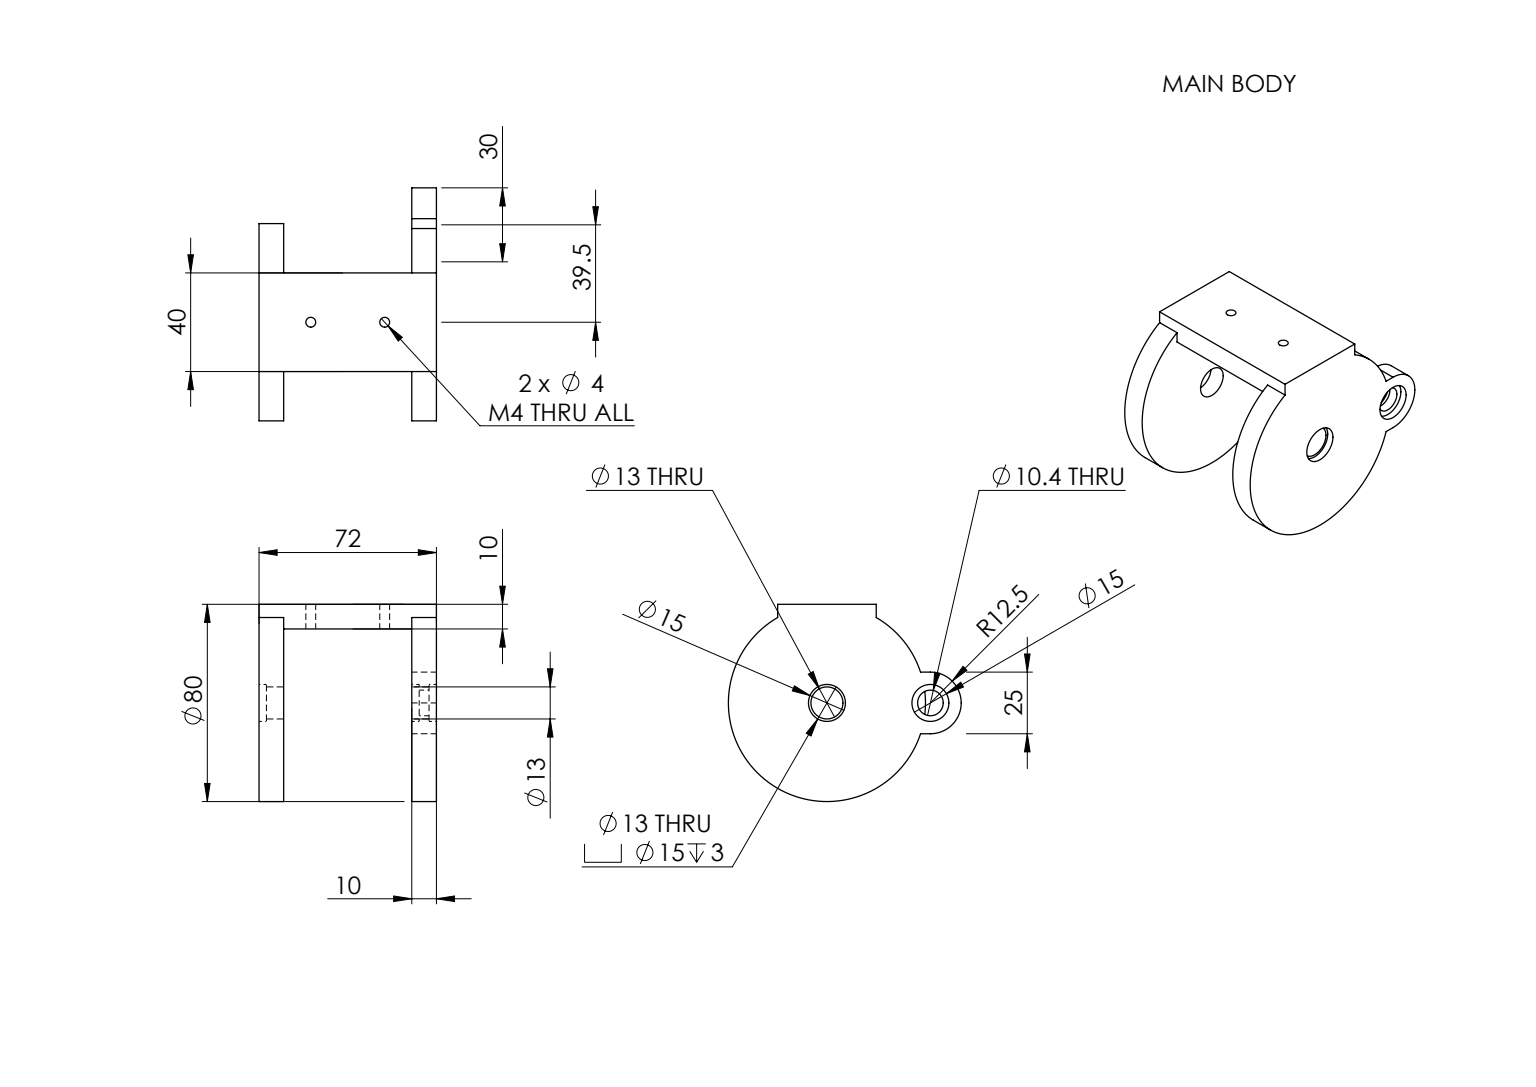
ISO-10303-21;
HEADER;
FILE_DESCRIPTION (('STEP AP214'),
    '1' );
FILE_NAME ('main body.step',
    '2026-10-27T08:02:39',
    ( '' ),
    ( '' ),
    'SwSTEP 2.0',
    'SolidWorks 2026',
    '' );
FILE_SCHEMA (( 'AUTOMOTIVE_DESIGN' ));
ENDSEC;

DATA;
#9=CARTESIAN_POINT ( 'NONE',  ( -36.00100000000000477, 0.000000000000000000, -41.99999999999999289 ) ) ;
#10=ORIENTED_EDGE ( 'NONE', *, *, #7633, .F. ) ;
#14=CIRCLE ( 'NONE', #9018, 40.00000000000000711 ) ;
#19=DIRECTION ( 'NONE',  ( -0.000000000000000000, 1.000000000000000000, -0.000000000000000000 ) ) ;
#37=VECTOR ( 'NONE', #10938, 1000.000000000000000 ) ;
#47=DIRECTION ( 'NONE',  ( 0.000000000000000000, 0.000000000000000000, -1.000000000000000000 ) ) ;
#57=ORIENTED_EDGE ( 'NONE', *, *, #11975, .F. ) ;
#92=DIRECTION ( 'NONE',  ( 1.000000000000000000, -0.000000000000000000, -0.000000000000000000 ) ) ;
#93=CARTESIAN_POINT ( 'NONE',  ( 26.00000000000000355, 0.000000000000000000, -41.99999999999999289 ) ) ;
#96=VECTOR ( 'NONE', #10392, 1000.000000000000000 ) ;
#100=PRODUCT_CONTEXT ( 'NONE', #11984, 'mechanical' ) ;
#103=VERTEX_POINT ( 'NONE', #3228 ) ;
#115=CARTESIAN_POINT ( 'NONE',  ( -26.00000000000000355, -4.898587196589413815E-15, -40.00000000000000711 ) ) ;
#131=CARTESIAN_POINT ( 'NONE',  ( 29.00000000000000000, 9.184850993605147944E-16, -49.49999999999999289 ) ) ;
#146=FACE_OUTER_BOUND ( 'NONE', #6316, .T. ) ;
#153=EDGE_LOOP ( 'NONE', ( #1044, #6924 ) ) ;
#162=DIRECTION ( 'NONE',  ( 1.000000000000000000, 0.000000000000000000, 0.000000000000000000 ) ) ;
#184=DIRECTION ( 'NONE',  ( 1.000000000000000000, 0.000000000000000000, 0.000000000000000000 ) ) ;
#188=CIRCLE ( 'NONE', #6974, 7.500000000000000888 ) ;
#197=CIRCLE ( 'NONE', #11173, 2.000000000000000000 ) ;
#203=CYLINDRICAL_SURFACE ( 'NONE', #8088, 7.500000000000000000 ) ;
#212=CARTESIAN_POINT ( 'NONE',  ( 0.000000000000000000, 0.000000000000000000, 0.000000000000000000 ) ) ;
#213=CIRCLE ( 'NONE', #1019, 7.500000000000000888 ) ;
#231=VERTEX_POINT ( 'NONE', #3477 ) ;
#248=ORIENTED_EDGE ( 'NONE', *, *, #430, .T. ) ;
#256=VECTOR ( 'NONE', #8139, 1000.000000000000000 ) ;
#257=AXIS2_PLACEMENT_3D ( 'NONE', #8422, #11402, #2776 ) ;
#264=ORIENTED_EDGE ( 'NONE', *, *, #11856, .T. ) ;
#278=FACE_OUTER_BOUND ( 'NONE', #10185, .T. ) ;
#294=DIRECTION ( 'NONE',  ( 0.000000000000000000, 0.000000000000000000, -1.000000000000000000 ) ) ;
#297=EDGE_LOOP ( 'NONE', ( #11234, #9949, #2749, #9847 ) ) ;
#298=ORIENTED_EDGE ( 'NONE', *, *, #9479, .T. ) ;
#303=VERTEX_POINT ( 'NONE', #4769 ) ;
#313=MANIFOLD_SOLID_BREP ( 'AdvancedHole1', #9575 ) ;
#315=DIRECTION ( 'NONE',  ( 0.000000000000000000, 0.000000000000000000, -1.000000000000000000 ) ) ;
#322=ORIENTED_EDGE ( 'NONE', *, *, #10069, .T. ) ;
#336=ADVANCED_FACE ( 'NONE', ( #548 ), #10928, .F. ) ;
#387=AXIS2_PLACEMENT_3D ( 'NONE', #11303, #6559, #3504 ) ;
#392=EDGE_LOOP ( 'NONE', ( #8569, #7501, #1729, #4037 ) ) ;
#396=EDGE_CURVE ( 'NONE', #709, #1692, #8083, .T. ) ;
#426=AXIS2_PLACEMENT_3D ( 'NONE', #93, #5779, #1149 ) ;
#429=DIRECTION ( 'NONE',  ( -1.000000000000000000, -0.000000000000000000, -0.000000000000000000 ) ) ;
#430=EDGE_CURVE ( 'NONE', #4941, #709, #2995, .T. ) ;
#433=CARTESIAN_POINT ( 'NONE',  ( 29.00000000000000000, 0.000000000000000000, -34.49999999999999289 ) ) ;
#442=CARTESIAN_POINT ( 'NONE',  ( -26.00000000000000355, 30.00000000000000711, 20.00000000000001066 ) ) ;
#447=EDGE_CURVE ( 'NONE', #1975, #4496, #2545, .T. ) ;
#451=VERTEX_POINT ( 'NONE', #614 ) ;
#483=CARTESIAN_POINT ( 'NONE',  ( 26.00000000000000355, -12.50000000000000000, -37.99671038392666134 ) ) ;
#491=ORIENTED_EDGE ( 'NONE', *, *, #2315, .T. ) ;
#506=SURFACE_STYLE_FILL_AREA ( #8323 ) ;
#508=ORIENTED_EDGE ( 'NONE', *, *, #2896, .F. ) ;
#510=ORIENTED_EDGE ( 'NONE', *, *, #3017, .F. ) ;
#516=CYLINDRICAL_SURFACE ( 'NONE', #1244, 40.00000000000000711 ) ;
#531=FACE_BOUND ( 'NONE', #11009, .T. ) ;
#532=ORIENTED_EDGE ( 'NONE', *, *, #567, .F. ) ;
#548=FACE_OUTER_BOUND ( 'NONE', #392, .T. ) ;
#550=DIRECTION ( 'NONE',  ( 0.000000000000000000, 0.000000000000000000, 1.000000000000000000 ) ) ;
#552=FACE_BOUND ( 'NONE', #153, .T. ) ;
#567=EDGE_CURVE ( 'NONE', #11902, #11981, #6636, .T. ) ;
#571=DIRECTION ( 'NONE',  ( 1.000000000000000000, -0.000000000000000000, -0.000000000000000000 ) ) ;
#572=AXIS2_PLACEMENT_3D ( 'NONE', #11910, #10065, #680 ) ;
#589=LINE ( 'NONE', #3484, #11033 ) ;
#591=CARTESIAN_POINT ( 'NONE',  ( 36.00000000000000711, 0.000000000000000000, -41.99999999999999289 ) ) ;
#596=AXIS2_PLACEMENT_3D ( 'NONE', #7195, #3371, #9943 ) ;
#598=CARTESIAN_POINT ( 'NONE',  ( 33.00000000000000000, 0.000000000000000000, 0.000000000000000000 ) ) ;
#603=AXIS2_PLACEMENT_3D ( 'NONE', #7936, #5992, #9880 ) ;
#614=CARTESIAN_POINT ( 'NONE',  ( 33.00000000000000000, 0.000000000000000000, -47.19999999999998863 ) ) ;
#657=DIRECTION ( 'NONE',  ( 1.000000000000000000, 0.000000000000000000, 0.000000000000000000 ) ) ;
#663=ADVANCED_FACE ( 'NONE', ( #9634 ), #5938, .T. ) ;
#664=DIRECTION ( 'NONE',  ( -0.000000000000000000, 1.000000000000000000, -0.000000000000000000 ) ) ;
#680=DIRECTION ( 'NONE',  ( 0.000000000000000000, 0.000000000000000000, -1.000000000000000000 ) ) ;
#682=CARTESIAN_POINT ( 'NONE',  ( 36.00000000000000711, 34.64101615137756340, -19.99999999999998934 ) ) ;
#688=DIRECTION ( 'NONE',  ( 0.000000000000000000, -0.000000000000000000, 1.000000000000000000 ) ) ;
#689=PLANE ( 'NONE',  #1651 ) ;
#691=ORIENTED_EDGE ( 'NONE', *, *, #7322, .T. ) ;
#704=LINE ( 'NONE', #8215, #4042 ) ;
#709=VERTEX_POINT ( 'NONE', #9052 ) ;
#726=CARTESIAN_POINT ( 'NONE',  ( 26.00000000000000355, 0.000000000000000000, 0.000000000000000000 ) ) ;
#735=ORIENTED_EDGE ( 'NONE', *, *, #8854, .T. ) ;
#739=FACE_OUTER_BOUND ( 'NONE', #4011, .T. ) ;
#741=EDGE_LOOP ( 'NONE', ( #2743, #11355 ) ) ;
#754=DIRECTION ( 'NONE',  ( -1.000000000000000000, -0.000000000000000000, -0.000000000000000000 ) ) ;
#755=ORIENTED_EDGE ( 'NONE', *, *, #1742, .T. ) ;
#780=FACE_OUTER_BOUND ( 'NONE', #2241, .T. ) ;
#790=EDGE_CURVE ( 'NONE', #1934, #9986, #4294, .T. ) ;
#794=FACE_OUTER_BOUND ( 'NONE', #9487, .T. ) ;
#807=EDGE_CURVE ( 'NONE', #5230, #2486, #7399, .T. ) ;
#825=VERTEX_POINT ( 'NONE', #483 ) ;
#829=EDGE_LOOP ( 'NONE', ( #5890, #10432, #3205, #5681, #3589, #1932, #7496, #8486 ) ) ;
#837=VECTOR ( 'NONE', #8894, 1000.000000000000000 ) ;
#842=DIRECTION ( 'NONE',  ( 1.000000000000000000, -0.000000000000000000, -0.000000000000000000 ) ) ;
#843=LINE ( 'NONE', #5480, #11789 ) ;
#844=ORIENTED_EDGE ( 'NONE', *, *, #6702, .F. ) ;
#903=DIRECTION ( 'NONE',  ( 1.000000000000000000, -0.000000000000000000, -0.000000000000000000 ) ) ;
#912=EDGE_LOOP ( 'NONE', ( #4953, #8523 ) ) ;
#921=DIRECTION ( 'NONE',  ( 1.000000000000000000, 0.000000000000000000, 0.000000000000000000 ) ) ;
#959=ORIENTED_EDGE ( 'NONE', *, *, #12102, .F. ) ;
#964=DIRECTION ( 'NONE',  ( 0.000000000000000000, 0.000000000000000000, 1.000000000000000000 ) ) ;
#969=CARTESIAN_POINT ( 'NONE',  ( 29.00000000000000000, 0.000000000000000000, -41.99999999999999289 ) ) ;
#971=VECTOR ( 'NONE', #6375, 1000.000000000000000 ) ;
#977=CARTESIAN_POINT ( 'NONE',  ( 33.00000000000000000, 0.000000000000000000, 0.000000000000000000 ) ) ;
#983=ORIENTED_EDGE ( 'NONE', *, *, #11550, .F. ) ;
#1000=CARTESIAN_POINT ( 'NONE',  ( 36.00000000000000711, 0.000000000000000000, 0.000000000000000000 ) ) ;
#1019=AXIS2_PLACEMENT_3D ( 'NONE', #11811, #1311, #7951 ) ;
#1035=VECTOR ( 'NONE', #1350, 1000.000000000000000 ) ;
#1044=ORIENTED_EDGE ( 'NONE', *, *, #4471, .F. ) ;
#1051=EDGE_CURVE ( 'NONE', #9332, #5880, #9739, .T. ) ;
#1065=DIRECTION ( 'NONE',  ( 0.000000000000000000, 0.000000000000000000, 1.000000000000000000 ) ) ;
#1089=AXIS2_PLACEMENT_3D ( 'NONE', #3095, #10765, #8031 ) ;
#1096=CIRCLE ( 'NONE', #10089, 12.49999999999999645 ) ;
#1126=CARTESIAN_POINT ( 'NONE',  ( 26.00000000000000355, 0.000000000000000000, -41.99999999999999289 ) ) ;
#1128=ORIENTED_EDGE ( 'NONE', *, *, #8084, .T. ) ;
#1149=DIRECTION ( 'NONE',  ( 0.000000000000000000, 0.000000000000000000, 1.000000000000000000 ) ) ;
#1151=ORIENTED_EDGE ( 'NONE', *, *, #2334, .F. ) ;
#1152=DIRECTION ( 'NONE',  ( 0.000000000000000000, 1.000000000000000000, 0.000000000000000000 ) ) ;
#1156=CARTESIAN_POINT ( 'NONE',  ( -26.00000000000000355, 0.000000000000000000, 0.000000000000000000 ) ) ;
#1164=AXIS2_PLACEMENT_3D ( 'NONE', #1603, #3421, #7254 ) ;
#1166=CIRCLE ( 'NONE', #8970, 12.49999999999999645 ) ;
#1198=DIRECTION ( 'NONE',  ( -0.000000000000000000, 1.000000000000000000, -0.000000000000000000 ) ) ;
#1215=CARTESIAN_POINT ( 'NONE',  ( 26.00000000000000355, 7.960204194457796463E-16, -6.500000000000000888 ) ) ;
#1218=VECTOR ( 'NONE', #8496, 1000.000000000000000 ) ;
#1220=ORIENTED_EDGE ( 'NONE', *, *, #12267, .F. ) ;
#1232=ORIENTED_EDGE ( 'NONE', *, *, #5271, .T. ) ;
#1244=AXIS2_PLACEMENT_3D ( 'NONE', #11020, #571, #5466 ) ;
#1248=LINE ( 'NONE', #5066, #837 ) ;
#1271=CARTESIAN_POINT ( 'NONE',  ( -36.00000000000000711, 0.000000000000000000, 0.000000000000000000 ) ) ;
#1288=CIRCLE ( 'NONE', #1089, 40.00000000000000711 ) ;
#1298=AXIS2_PLACEMENT_3D ( 'NONE', #8826, #184, #9826 ) ;
#1299=CARTESIAN_POINT ( 'NONE',  ( 33.00000000000000000, 9.184850993605149917E-16, 7.500000000000000888 ) ) ;
#1304=CARTESIAN_POINT ( 'NONE',  ( -36.00000000000000000, 40.00000000000000711, 20.00000000000001066 ) ) ;
#1311=DIRECTION ( 'NONE',  ( 1.000000000000000000, 0.000000000000000000, 0.000000000000000000 ) ) ;
#1315=EDGE_LOOP ( 'NONE', ( #8246, #5545, #4189, #9435 ) ) ;
#1317=EDGE_CURVE ( 'NONE', #2662, #10589, #3298, .T. ) ;
#1320=VERTEX_POINT ( 'NONE', #4590 ) ;
#1325=CARTESIAN_POINT ( 'NONE',  ( -36.00000000000000711, 0.000000000000000000, 6.500000000000000888 ) ) ;
#1328=CARTESIAN_POINT ( 'NONE',  ( 26.00000000000000355, 12.50000000000000000, -24.50000000000000000 ) ) ;
#1329=ORIENTED_EDGE ( 'NONE', *, *, #10497, .T. ) ;
#1331=CARTESIAN_POINT ( 'NONE',  ( -26.00000000000000355, 34.64101615137756340, -19.99999999999998934 ) ) ;
#1341=CARTESIAN_POINT ( 'NONE',  ( -15.00000000000000000, 40.00000000000000711, -2.000000000000000000 ) ) ;
#1350=DIRECTION ( 'NONE',  ( 1.000000000000000000, -0.000000000000000000, -0.000000000000000000 ) ) ;
#1363=LINE ( 'NONE', #433, #6985 ) ;
#1395=ORIENTED_EDGE ( 'NONE', *, *, #8716, .F. ) ;
#1397=EDGE_CURVE ( 'NONE', #8903, #2114, #6531, .T. ) ;
#1417=CIRCLE ( 'NONE', #11191, 40.00000000000000711 ) ;
#1424=VERTEX_POINT ( 'NONE', #11327 ) ;
#1427=COLOUR_RGB ( '',0.8941176470588234615, 0.8941176470588234615, 0.8941176470588234615 ) ;
#1434=CARTESIAN_POINT ( 'NONE',  ( -36.00000000000000711, 34.64101615137756340, -19.99999999999998934 ) ) ;
#1437=ADVANCED_FACE ( 'NONE', ( #10586, #10331 ), #8536, .T. ) ;
#1447=LINE ( 'NONE', #442, #256 ) ;
#1468=CARTESIAN_POINT ( 'NONE',  ( 36.00000000000000000, 30.00000000000000711, -19.99999999999998934 ) ) ;
#1478=DIRECTION ( 'NONE',  ( -1.000000000000000000, 0.000000000000000000, 0.000000000000000000 ) ) ;
#1485=ADVANCED_FACE ( 'NONE', ( #146 ), #1910, .F. ) ;
#1489=LINE ( 'NONE', #9124, #6369 ) ;
#1491=VERTEX_POINT ( 'NONE', #7725 ) ;
#1494=VERTEX_POINT ( 'NONE', #6594 ) ;
#1504=CARTESIAN_POINT ( 'NONE',  ( 29.00000000000000000, 0.000000000000000000, -41.99999999999999289 ) ) ;
#1505=DIRECTION ( 'NONE',  ( 1.000000000000000000, 0.000000000000000000, 0.000000000000000000 ) ) ;
#1511=CARTESIAN_POINT ( 'NONE',  ( 26.00000000000000355, 0.000000000000000000, 0.000000000000000000 ) ) ;
#1521=CARTESIAN_POINT ( 'NONE',  ( 36.00000000000000711, 0.000000000000000000, 40.00000000000000711 ) ) ;
#1522=LINE ( 'NONE', #9285, #12208 ) ;
#1535=DIRECTION ( 'NONE',  ( -0.000000000000000000, 1.000000000000000000, 0.000000000000000000 ) ) ;
#1542=ORIENTED_EDGE ( 'NONE', *, *, #447, .F. ) ;
#1547=ORIENTED_EDGE ( 'NONE', *, *, #4092, .F. ) ;
#1550=ORIENTED_EDGE ( 'NONE', *, *, #10879, .T. ) ;
#1571=EDGE_CURVE ( 'NONE', #9332, #4951, #6562, .T. ) ;
#1589=CARTESIAN_POINT ( 'NONE',  ( 26.00000000000000355, 34.64101615137754919, 20.00000000000000711 ) ) ;
#1594=FACE_OUTER_BOUND ( 'NONE', #8873, .T. ) ;
#1603=CARTESIAN_POINT ( 'NONE',  ( -13.05124837953327344, 0.000000000000000000, -41.99999999999999289 ) ) ;
#1605=ORIENTED_EDGE ( 'NONE', *, *, #9074, .T. ) ;
#1637=AXIS2_PLACEMENT_3D ( 'NONE', #7596, #92, #6914 ) ;
#1639=AXIS2_PLACEMENT_3D ( 'NONE', #1955, #4829, #8652 ) ;
#1651=AXIS2_PLACEMENT_3D ( 'NONE', #7383, #12110, #6376 ) ;
#1655=UNCERTAINTY_MEASURE_WITH_UNIT (LENGTH_MEASURE( 1.000000000000000082E-05 ), #6454, 'distance_accuracy_value', 'NONE');
#1665=CARTESIAN_POINT ( 'NONE',  ( 28.99999999999999645, 6.368163355566238354E-16, -36.79999999999999716 ) ) ;
#1684=CARTESIAN_POINT ( 'NONE',  ( -36.00100000000000477, 0.000000000000000000, -47.19999999999998863 ) ) ;
#1686=VERTEX_POINT ( 'NONE', #3101 ) ;
#1692=VERTEX_POINT ( 'NONE', #2092 ) ;
#1694=( NAMED_UNIT ( * ) PLANE_ANGLE_UNIT ( ) SI_UNIT ( $, .RADIAN. ) );
#1697=ORIENTED_EDGE ( 'NONE', *, *, #7444, .T. ) ;
#1709=VERTEX_POINT ( 'NONE', #9858 ) ;
#1721=ORIENTED_EDGE ( 'NONE', *, *, #7312, .T. ) ;
#1729=ORIENTED_EDGE ( 'NONE', *, *, #7563, .F. ) ;
#1742=EDGE_CURVE ( 'NONE', #8475, #303, #4087, .T. ) ;
#1752=CARTESIAN_POINT ( 'NONE',  ( 26.00000000000000355, 0.000000000000000000, -41.99999999999999289 ) ) ;
#1758=ORIENTED_EDGE ( 'NONE', *, *, #10893, .F. ) ;
#1761=ORIENTED_EDGE ( 'NONE', *, *, #2117, .F. ) ;
#1776=CARTESIAN_POINT ( 'NONE',  ( 36.00000000000000711, 0.000000000000000000, 0.000000000000000000 ) ) ;
#1790=FACE_BOUND ( 'NONE', #2715, .T. ) ;
#1796=DIRECTION ( 'NONE',  ( 0.000000000000000000, 0.000000000000000000, 1.000000000000000000 ) ) ;
#1806=DIRECTION ( 'NONE',  ( 1.000000000000000000, -0.000000000000000000, -0.000000000000000000 ) ) ;
#1810=DIRECTION ( 'NONE',  ( -0.000000000000000000, 1.000000000000000000, 0.000000000000000000 ) ) ;
#1813=ORIENTED_EDGE ( 'NONE', *, *, #6114, .F. ) ;
#1825=AXIS2_PLACEMENT_3D ( 'NONE', #7929, #9873, #6296 ) ;
#1838=ORIENTED_EDGE ( 'NONE', *, *, #396, .T. ) ;
#1840=CIRCLE ( 'NONE', #2837, 7.500000000000000000 ) ;
#1861=AXIS2_PLACEMENT_3D ( 'NONE', #4094, #10529, #7862 ) ;
#1863=CARTESIAN_POINT ( 'NONE',  ( 26.00000000000000355, 0.000000000000000000, 0.000000000000000000 ) ) ;
#1869=ADVANCED_FACE ( 'NONE', ( #5394 ), #11081, .F. ) ;
#1872=DIRECTION ( 'NONE',  ( 0.000000000000000000, 0.000000000000000000, -1.000000000000000000 ) ) ;
#1874=EDGE_LOOP ( 'NONE', ( #1935, #4316, #491, #959 ) ) ;
#1877=DIRECTION ( 'NONE',  ( 1.000000000000000000, -0.000000000000000000, -0.000000000000000000 ) ) ;
#1878=CARTESIAN_POINT ( 'NONE',  ( 36.00000000000000711, 0.000000000000000000, 0.000000000000000000 ) ) ;
#1910=PLANE ( 'NONE',  #2966 ) ;
#1925=FACE_BOUND ( 'NONE', #6583, .T. ) ;
#1932=ORIENTED_EDGE ( 'NONE', *, *, #3099, .T. ) ;
#1934=VERTEX_POINT ( 'NONE', #6518 ) ;
#1935=ORIENTED_EDGE ( 'NONE', *, *, #12053, .F. ) ;
#1938=CARTESIAN_POINT ( 'NONE',  ( -36.00100000000000477, 0.000000000000000000, -41.99999999999999289 ) ) ;
#1941=CARTESIAN_POINT ( 'NONE',  ( 26.00000000000000355, 0.000000000000000000, 6.500000000000000888 ) ) ;
#1955=CARTESIAN_POINT ( 'NONE',  ( -13.05124837953327344, -12.50000000000000000, -24.50000000000000000 ) ) ;
#1975=VERTEX_POINT ( 'NONE', #10511 ) ;
#2015=AXIS2_PLACEMENT_3D ( 'NONE', #4944, #11557, #3087 ) ;
#2033=DIRECTION ( 'NONE',  ( 0.000000000000000000, 0.000000000000000000, -1.000000000000000000 ) ) ;
#2053=DIRECTION ( 'NONE',  ( 1.000000000000000000, -0.000000000000000000, -0.000000000000000000 ) ) ;
#2056=DIRECTION ( 'NONE',  ( 1.000000000000000000, -0.000000000000000000, -0.000000000000000000 ) ) ;
#2062=DIRECTION ( 'NONE',  ( 1.000000000000000000, 0.000000000000000000, -0.000000000000000000 ) ) ;
#2073=CYLINDRICAL_SURFACE ( 'NONE', #12012, 7.500000000000000888 ) ;
#2082=CARTESIAN_POINT ( 'NONE',  ( -36.00000000000000711, -9.184850993605149917E-16, 7.500000000000000888 ) ) ;
#2085=CYLINDRICAL_SURFACE ( 'NONE', #4823, 5.199999999999996625 ) ;
#2092=CARTESIAN_POINT ( 'NONE',  ( 36.00000000000000711, 0.000000000000000000, -49.49999999999999289 ) ) ;
#2108=FACE_OUTER_BOUND ( 'NONE', #4777, .T. ) ;
#2109=ORIENTED_EDGE ( 'NONE', *, *, #10098, .T. ) ;
#2114=VERTEX_POINT ( 'NONE', #4185 ) ;
#2117=EDGE_CURVE ( 'NONE', #1320, #10764, #7211, .T. ) ;
#2129=ORIENTED_EDGE ( 'NONE', *, *, #1571, .F. ) ;
#2140=EDGE_CURVE ( 'NONE', #1975, #825, #8952, .T. ) ;
#2147=VERTEX_POINT ( 'NONE', #9768 ) ;
#2157=FACE_OUTER_BOUND ( 'NONE', #6571, .T. ) ;
#2159=ORIENTED_EDGE ( 'NONE', *, *, #4246, .T. ) ;
#2160=ORIENTED_EDGE ( 'NONE', *, *, #11856, .F. ) ;
#2166=ORIENTED_EDGE ( 'NONE', *, *, #2958, .T. ) ;
#2173=ADVANCED_FACE ( 'NONE', ( #11347, #10011 ), #2366, .T. ) ;
#2182=ADVANCED_FACE ( 'NONE', ( #10930 ), #4253, .F. ) ;
#2190=LINE ( 'NONE', #6129, #10988 ) ;
#2241=EDGE_LOOP ( 'NONE', ( #1761, #9174, #4530, #6960 ) ) ;
#2243=CARTESIAN_POINT ( 'NONE',  ( 36.00000000000000711, 0.000000000000000000, -54.50000000000000000 ) ) ;
#2249=ORIENTED_EDGE ( 'NONE', *, *, #10231, .T. ) ;
#2252=VECTOR ( 'NONE', #11067, 1000.000000000000000 ) ;
#2281=CIRCLE ( 'NONE', #7082, 1.999999999999998224 ) ;
#2298=VERTEX_POINT ( 'NONE', #8617 ) ;
#2303=LINE ( 'NONE', #1434, #5639 ) ;
#2311=FACE_BOUND ( 'NONE', #10416, .T. ) ;
#2315=EDGE_CURVE ( 'NONE', #2452, #10319, #7420, .T. ) ;
#2334=EDGE_CURVE ( 'NONE', #1494, #3376, #2866, .T. ) ;
#2354=ADVANCED_FACE ( 'NONE', ( #3923, #2108 ), #9552, .T. ) ;
#2362=CARTESIAN_POINT ( 'NONE',  ( 26.00000000000000355, 12.50000000000000000, -41.99999999999999289 ) ) ;
#2366=PLANE ( 'NONE',  #2407 ) ;
#2383=CIRCLE ( 'NONE', #7794, 12.49999999999999645 ) ;
#2386=CIRCLE ( 'NONE', #5753, 7.500000000000000888 ) ;
#2392=CYLINDRICAL_SURFACE ( 'NONE', #5568, 7.500000000000000000 ) ;
#2394=ORIENTED_EDGE ( 'NONE', *, *, #8102, .F. ) ;
#2400=CARTESIAN_POINT ( 'NONE',  ( -15.00000000000000000, 30.00000000000000711, 0.000000000000000000 ) ) ;
#2407=AXIS2_PLACEMENT_3D ( 'NONE', #1504, #11118, #550 ) ;
#2418=AXIS2_PLACEMENT_3D ( 'NONE', #977, #921, #47 ) ;
#2422=EDGE_CURVE ( 'NONE', #303, #11981, #4418, .T. ) ;
#2426=VERTEX_POINT ( 'NONE', #12345 ) ;
#2429=CYLINDRICAL_SURFACE ( 'NONE', #9502, 7.500000000000000000 ) ;
#2432=EDGE_CURVE ( 'NONE', #6862, #5581, #14, .T. ) ;
#2440=LINE ( 'NONE', #8318, #2252 ) ;
#2450=CIRCLE ( 'NONE', #6624, 5.199999999999996625 ) ;
#2452=VERTEX_POINT ( 'NONE', #1341 ) ;
#2457=CIRCLE ( 'NONE', #6260, 7.500000000000000000 ) ;
#2461=CARTESIAN_POINT ( 'NONE',  ( -13.05124837953327344, 12.50000000000000000, -41.99999999999999289 ) ) ;
#2463=ORIENTED_EDGE ( 'NONE', *, *, #7322, .F. ) ;
#2479=ORIENTED_EDGE ( 'NONE', *, *, #7267, .F. ) ;
#2482=CARTESIAN_POINT ( 'NONE',  ( 36.00000000000000000, 40.00000000000000711, 20.00000000000001066 ) ) ;
#2486=VERTEX_POINT ( 'NONE', #10786 ) ;
#2545=LINE ( 'NONE', #3558, #10976 ) ;
#2547=DIRECTION ( 'NONE',  ( -0.000000000000000000, 1.000000000000000000, -0.000000000000000000 ) ) ;
#2548=EDGE_CURVE ( 'NONE', #4639, #4147, #10908, .T. ) ;
#2551=DIRECTION ( 'NONE',  ( 1.000000000000000000, -0.000000000000000000, -0.000000000000000000 ) ) ;
#2552=ADVANCED_FACE ( 'NONE', ( #531, #2157 ), #5048, .T. ) ;
#2553=EDGE_LOOP ( 'NONE', ( #8988, #1128, #7779, #7206, #2918, #2166, #691, #2249, #9046, #2109 ) ) ;
#2556=( LENGTH_UNIT ( ) NAMED_UNIT ( * ) SI_UNIT ( .MILLI., .METRE. ) );
#2567=DIRECTION ( 'NONE',  ( 0.000000000000000000, -0.000000000000000000, 1.000000000000000000 ) ) ;
#2570=APPLICATION_CONTEXT ( 'automotive_design' ) ;
#2581=EDGE_CURVE ( 'NONE', #6339, #1692, #5417, .T. ) ;
#2625=( NAMED_UNIT ( * ) SI_UNIT ( $, .STERADIAN. ) SOLID_ANGLE_UNIT ( ) );
#2629=EDGE_LOOP ( 'NONE', ( #11526, #3927, #5490, #12163 ) ) ;
#2641=FACE_OUTER_BOUND ( 'NONE', #297, .T. ) ;
#2642=AXIS2_PLACEMENT_3D ( 'NONE', #1000, #9706, #8757 ) ;
#2651=EDGE_CURVE ( 'NONE', #2486, #4605, #843, .T. ) ;
#2659=LINE ( 'NONE', #5589, #9831 ) ;
#2661=VERTEX_POINT ( 'NONE', #1665 ) ;
#2662=VERTEX_POINT ( 'NONE', #9300 ) ;
#2675=DIRECTION ( 'NONE',  ( 1.000000000000000000, 0.000000000000000000, 0.000000000000000000 ) ) ;
#2676=ORIENTED_EDGE ( 'NONE', *, *, #2117, .T. ) ;
#2688=ORIENTED_EDGE ( 'NONE', *, *, #7992, .T. ) ;
#2715=EDGE_LOOP ( 'NONE', ( #9455, #9983 ) ) ;
#2722=DIRECTION ( 'NONE',  ( 1.000000000000000000, 0.000000000000000000, 0.000000000000000000 ) ) ;
#2743=ORIENTED_EDGE ( 'NONE', *, *, #8913, .T. ) ;
#2748=DIRECTION ( 'NONE',  ( -1.000000000000000000, -0.000000000000000000, -0.000000000000000000 ) ) ;
#2749=ORIENTED_EDGE ( 'NONE', *, *, #10679, .F. ) ;
#2758=CARTESIAN_POINT ( 'NONE',  ( -33.00000000000000000, 0.000000000000000000, 0.000000000000000000 ) ) ;
#2764=EDGE_LOOP ( 'NONE', ( #1329, #2839 ) ) ;
#2776=DIRECTION ( 'NONE',  ( 0.000000000000000000, 0.000000000000000000, 1.000000000000000000 ) ) ;
#2803=EDGE_CURVE ( 'NONE', #1424, #1709, #5830, .T. ) ;
#2821=AXIS2_PLACEMENT_3D ( 'NONE', #4721, #664, #7600 ) ;
#2834=AXIS2_PLACEMENT_3D ( 'NONE', #1776, #9482, #5412 ) ;
#2836=DIRECTION ( 'NONE',  ( 0.000000000000000000, 0.000000000000000000, -1.000000000000000000 ) ) ;
#2837=AXIS2_PLACEMENT_3D ( 'NONE', #1126, #10446, #4937 ) ;
#2838=VECTOR ( 'NONE', #10774, 1000.000000000000000 ) ;
#2839=ORIENTED_EDGE ( 'NONE', *, *, #4092, .T. ) ;
#2844=CARTESIAN_POINT ( 'NONE',  ( -33.00000000000000000, 0.000000000000000000, 6.500000000000000888 ) ) ;
#2851=CYLINDRICAL_SURFACE ( 'NONE', #257, 6.500000000000000888 ) ;
#2866=LINE ( 'NONE', #3979, #11990 ) ;
#2877=CARTESIAN_POINT ( 'NONE',  ( 15.00000000000000355, 40.00000000000000711, 1.999999999999998224 ) ) ;
#2887=FACE_OUTER_BOUND ( 'NONE', #5644, .T. ) ;
#2890=DIRECTION ( 'NONE',  ( 0.000000000000000000, 0.000000000000000000, -1.000000000000000000 ) ) ;
#2896=EDGE_CURVE ( 'NONE', #1494, #9332, #8834, .T. ) ;
#2900=DIRECTION ( 'NONE',  ( 0.000000000000000000, 0.000000000000000000, 1.000000000000000000 ) ) ;
#2918=ORIENTED_EDGE ( 'NONE', *, *, #2432, .T. ) ;
#2923=CARTESIAN_POINT ( 'NONE',  ( 33.00000000000000000, 0.000000000000000000, -41.99999999999999289 ) ) ;
#2924=DIRECTION ( 'NONE',  ( 0.000000000000000000, 0.000000000000000000, -1.000000000000000000 ) ) ;
#2935=ADVANCED_FACE ( 'NONE', ( #278 ), #9789, .F. ) ;
#2936=FACE_BOUND ( 'NONE', #912, .T. ) ;
#2939=CARTESIAN_POINT ( 'NONE',  ( 26.00000000000000355, 0.000000000000000000, 0.000000000000000000 ) ) ;
#2941=CYLINDRICAL_SURFACE ( 'NONE', #6493, 6.500000000000000888 ) ;
#2958=EDGE_CURVE ( 'NONE', #5581, #10639, #4203, .T. ) ;
#2966=AXIS2_PLACEMENT_3D ( 'NONE', #12321, #10399, #11576 ) ;
#2995=CIRCLE ( 'NONE', #387, 7.500000000000000000 ) ;
#3014=CARTESIAN_POINT ( 'NONE',  ( -26.00000000000000355, 30.00000000000000711, 20.00000000000001066 ) ) ;
#3017=EDGE_CURVE ( 'NONE', #8676, #6734, #3104, .T. ) ;
#3024=ORIENTED_EDGE ( 'NONE', *, *, #4423, .F. ) ;
#3062=AXIS2_PLACEMENT_3D ( 'NONE', #11201, #7341, #2567 ) ;
#3085=LINE ( 'NONE', #9764, #8389 ) ;
#3087=DIRECTION ( 'NONE',  ( 0.000000000000000000, 0.000000000000000000, 1.000000000000000000 ) ) ;
#3093=CARTESIAN_POINT ( 'NONE',  ( -15.00000000000000000, 40.00000000000000711, 0.000000000000000000 ) ) ;
#3094=ORIENTED_EDGE ( 'NONE', *, *, #2896, .T. ) ;
#3095=CARTESIAN_POINT ( 'NONE',  ( -26.00000000000000355, 0.000000000000000000, 0.000000000000000000 ) ) ;
#3099=EDGE_CURVE ( 'NONE', #5581, #12066, #6338, .T. ) ;
#3101=CARTESIAN_POINT ( 'NONE',  ( 36.00000000000000711, 9.184850993605149917E-16, 7.500000000000000888 ) ) ;
#3104=LINE ( 'NONE', #1328, #4219 ) ;
#3120=CARTESIAN_POINT ( 'NONE',  ( -15.00000000000000000, 40.00000000000000711, 0.000000000000000000 ) ) ;
#3130=PRODUCT_DEFINITION ( 'UNKNOWN', '', #10232, #9902 ) ;
#3131=ORIENTED_EDGE ( 'NONE', *, *, #8782, .T. ) ;
#3163=EDGE_CURVE ( 'NONE', #9430, #1491, #1522, .T. ) ;
#3173=ADVANCED_FACE ( 'NONE', ( #2641 ), #516, .T. ) ;
#3176=CIRCLE ( 'NONE', #6764, 40.00000000000000711 ) ;
#3183=AXIS2_PLACEMENT_3D ( 'NONE', #1863, #9492, #4674 ) ;
#3190=CARTESIAN_POINT ( 'NONE',  ( -33.00000000000000000, -7.960204194457796463E-16, -6.500000000000000888 ) ) ;
#3192=EDGE_CURVE ( 'NONE', #6862, #8676, #704, .T. ) ;
#3204=ORIENTED_EDGE ( 'NONE', *, *, #5271, .F. ) ;
#3205=ORIENTED_EDGE ( 'NONE', *, *, #4499, .T. ) ;
#3208=DIRECTION ( 'NONE',  ( 1.000000000000000000, 0.000000000000000000, 0.000000000000000000 ) ) ;
#3210=( GEOMETRIC_REPRESENTATION_CONTEXT ( 3 ) GLOBAL_UNCERTAINTY_ASSIGNED_CONTEXT ( ( #7792 ) ) GLOBAL_UNIT_ASSIGNED_CONTEXT ( ( #10329, #3718, #7530 ) ) REPRESENTATION_CONTEXT ( 'NONE', 'WORKASPACE' ) );
#3228=CARTESIAN_POINT ( 'NONE',  ( 26.00000000000000355, 30.00000000000000711, -19.99999999999998934 ) ) ;
#3238=CYLINDRICAL_SURFACE ( 'NONE', #11617, 12.49999999999999645 ) ;
#3241=EDGE_LOOP ( 'NONE', ( #6976, #6122 ) ) ;
#3275=ORIENTED_EDGE ( 'NONE', *, *, #10679, .T. ) ;
#3278=CIRCLE ( 'NONE', #5474, 7.500000000000000000 ) ;
#3288=DIRECTION ( 'NONE',  ( -1.000000000000000000, 0.000000000000000000, 0.000000000000000000 ) ) ;
#3297=DIRECTION ( 'NONE',  ( -0.000000000000000000, 1.000000000000000000, 0.000000000000000000 ) ) ;
#3298=LINE ( 'NONE', #6293, #9608 ) ;
#3302=ORIENTED_EDGE ( 'NONE', *, *, #10428, .T. ) ;
#3325=CARTESIAN_POINT ( 'NONE',  ( 26.00000000000000355, 30.00000000000000711, 0.000000000000000000 ) ) ;
#3328=CARTESIAN_POINT ( 'NONE',  ( 15.00000000000000355, 30.00000000000000711, 0.000000000000000000 ) ) ;
#3331=CARTESIAN_POINT ( 'NONE',  ( 33.00000000000000000, 9.184850993605147944E-16, -34.49999999999999289 ) ) ;
#3334=CARTESIAN_POINT ( 'NONE',  ( 36.00000000000000711, 9.184850993605147944E-16, -34.49999999999999289 ) ) ;
#3352=ORIENTED_EDGE ( 'NONE', *, *, #1317, .T. ) ;
#3354=ADVANCED_FACE ( 'NONE', ( #10648 ), #6769, .T. ) ;
#3355=VERTEX_POINT ( 'NONE', #3897 ) ;
#3365=VECTOR ( 'NONE', #11829, 1000.000000000000000 ) ;
#3371=DIRECTION ( 'NONE',  ( -1.000000000000000000, 0.000000000000000000, 0.000000000000000000 ) ) ;
#3374=FACE_BOUND ( 'NONE', #12099, .T. ) ;
#3376=VERTEX_POINT ( 'NONE', #7017 ) ;
#3398=ORIENTED_EDGE ( 'NONE', *, *, #11192, .F. ) ;
#3411=EDGE_CURVE ( 'NONE', #103, #2147, #5129, .T. ) ;
#3421=DIRECTION ( 'NONE',  ( 1.000000000000000000, 0.000000000000000000, 0.000000000000000000 ) ) ;
#3422=AXIS2_PLACEMENT_3D ( 'NONE', #2923, #5980, #5926 ) ;
#3448=FACE_OUTER_BOUND ( 'NONE', #5110, .T. ) ;
#3450=VERTEX_POINT ( 'NONE', #2082 ) ;
#3453=SURFACE_SIDE_STYLE ('',( #506 ) ) ;
#3455=AXIS2_PLACEMENT_3D ( 'NONE', #8022, #11001, #10931 ) ;
#3465=FACE_OUTER_BOUND ( 'NONE', #1315, .T. ) ;
#3468=ORIENTED_EDGE ( 'NONE', *, *, #2140, .T. ) ;
#3477=CARTESIAN_POINT ( 'NONE',  ( -33.00000000000000000, -9.184850993605149917E-16, 7.500000000000000888 ) ) ;
#3480=CARTESIAN_POINT ( 'NONE',  ( -36.00000000000000711, -4.898587196589413815E-15, -40.00000000000000711 ) ) ;
#3484=CARTESIAN_POINT ( 'NONE',  ( -15.00000000000000000, 40.00000000000000711, 2.000000000000000000 ) ) ;
#3498=EDGE_LOOP ( 'NONE', ( #6299, #5712, #9511, #7126 ) ) ;
#3504=DIRECTION ( 'NONE',  ( 0.000000000000000000, 0.000000000000000000, -1.000000000000000000 ) ) ;
#3507=CARTESIAN_POINT ( 'NONE',  ( -13.05124837953327344, 12.50000000000000000, -24.50000000000000000 ) ) ;
#3554=ADVANCED_FACE ( 'NONE', ( #12171, #552, #7329 ), #689, .F. ) ;
#3558=CARTESIAN_POINT ( 'NONE',  ( -13.05124837953327344, -12.50000000000000000, -41.99999999999999289 ) ) ;
#3564=ORIENTED_EDGE ( 'NONE', *, *, #10497, .F. ) ;
#3575=CIRCLE ( 'NONE', #9963, 6.500000000000000888 ) ;
#3578=EDGE_CURVE ( 'NONE', #8475, #11902, #4653, .T. ) ;
#3589=ORIENTED_EDGE ( 'NONE', *, *, #2958, .F. ) ;
#3614=CARTESIAN_POINT ( 'NONE',  ( 29.00000000000000000, 0.000000000000000000, -34.49999999999999289 ) ) ;
#3667=ORIENTED_EDGE ( 'NONE', *, *, #1571, .T. ) ;
#3671=CIRCLE ( 'NONE', #5876, 6.500000000000000888 ) ;
#3675=DIRECTION ( 'NONE',  ( -0.000000000000000000, -1.000000000000000000, -0.000000000000000000 ) ) ;
#3686=AXIS2_PLACEMENT_3D ( 'NONE', #5015, #11751, #9721 ) ;
#3691=DIRECTION ( 'NONE',  ( -0.000000000000000000, 1.000000000000000000, 0.000000000000000000 ) ) ;
#3698=DIRECTION ( 'NONE',  ( -1.000000000000000000, -0.000000000000000000, -0.000000000000000000 ) ) ;
#3704=CARTESIAN_POINT ( 'NONE',  ( 26.00000000000000355, 12.50000000000000000, -37.99671038392666134 ) ) ;
#3712=LINE ( 'NONE', #7346, #8224 ) ;
#3718=( NAMED_UNIT ( * ) PLANE_ANGLE_UNIT ( ) SI_UNIT ( $, .RADIAN. ) );
#3720=DIRECTION ( 'NONE',  ( 0.000000000000000000, 0.000000000000000000, 1.000000000000000000 ) ) ;
#3725=DIRECTION ( 'NONE',  ( 1.000000000000000000, -0.000000000000000000, -0.000000000000000000 ) ) ;
#3761=VERTEX_POINT ( 'NONE', #1941 ) ;
#3789=LINE ( 'NONE', #5542, #8364 ) ;
#3828=CIRCLE ( 'NONE', #10806, 6.500000000000000888 ) ;
#3840=AXIS2_PLACEMENT_3D ( 'NONE', #3093, #1198, #6906 ) ;
#3882=CARTESIAN_POINT ( 'NONE',  ( -36.00000000000000711, -7.960204194457796463E-16, -6.500000000000000888 ) ) ;
#3891=ORIENTED_EDGE ( 'NONE', *, *, #7693, .T. ) ;
#3897=CARTESIAN_POINT ( 'NONE',  ( -36.00000000000000000, 40.00000000000000711, -19.99999999999998934 ) ) ;
#3900=EDGE_CURVE ( 'NONE', #3355, #9986, #3938, .T. ) ;
#3923=FACE_BOUND ( 'NONE', #3241, .T. ) ;
#3927=ORIENTED_EDGE ( 'NONE', *, *, #6075, .T. ) ;
#3938=LINE ( 'NONE', #1304, #9067 ) ;
#3940=EDGE_LOOP ( 'NONE', ( #5628, #9952 ) ) ;
#3945=DIRECTION ( 'NONE',  ( -1.000000000000000000, -0.000000000000000000, -0.000000000000000000 ) ) ;
#3964=AXIS2_PLACEMENT_3D ( 'NONE', #5168, #6816, #2062 ) ;
#3966=CYLINDRICAL_SURFACE ( 'NONE', #1861, 40.00000000000000711 ) ;
#3969=CARTESIAN_POINT ( 'NONE',  ( 36.00000000000000711, -12.50000000000000000, -41.99999999999999289 ) ) ;
#3971=VERTEX_POINT ( 'NONE', #11071 ) ;
#3978=DIRECTION ( 'NONE',  ( -0.000000000000000000, 1.000000000000000000, 0.000000000000000000 ) ) ;
#3979=CARTESIAN_POINT ( 'NONE',  ( -36.00000000000000711, 0.000000000000000000, 40.00000000000000711 ) ) ;
#3982=CIRCLE ( 'NONE', #6796, 2.000000000000000000 ) ;
#3996=ORIENTED_EDGE ( 'NONE', *, *, #8102, .T. ) ;
#4001=DIRECTION ( 'NONE',  ( -1.000000000000000000, -0.000000000000000000, -0.000000000000000000 ) ) ;
#4002=VECTOR ( 'NONE', #7635, 1000.000000000000000 ) ;
#4011=EDGE_LOOP ( 'NONE', ( #1395, #7718, #510, #9691 ) ) ;
#4014=EDGE_LOOP ( 'NONE', ( #4354, #248 ) ) ;
#4021=EDGE_CURVE ( 'NONE', #10764, #1320, #2457, .T. ) ;
#4035=DIRECTION ( 'NONE',  ( 0.000000000000000000, 0.000000000000000000, 1.000000000000000000 ) ) ;
#4037=ORIENTED_EDGE ( 'NONE', *, *, #2548, .F. ) ;
#4042=VECTOR ( 'NONE', #754, 1000.000000000000000 ) ;
#4049=VERTEX_POINT ( 'NONE', #5325 ) ;
#4069=LINE ( 'NONE', #8947, #7300 ) ;
#4072=FACE_OUTER_BOUND ( 'NONE', #10061, .T. ) ;
#4075=VECTOR ( 'NONE', #8602, 1000.000000000000000 ) ;
#4078=ORIENTED_EDGE ( 'NONE', *, *, #5482, .T. ) ;
#4087=LINE ( 'NONE', #1325, #3365 ) ;
#4092=EDGE_CURVE ( 'NONE', #9430, #6597, #11238, .T. ) ;
#4094=CARTESIAN_POINT ( 'NONE',  ( -36.00000000000000711, 0.000000000000000000, 0.000000000000000000 ) ) ;
#4108=EDGE_LOOP ( 'NONE', ( #3094, #11544, #10303, #1151 ) ) ;
#4113=EDGE_LOOP ( 'NONE', ( #3996, #10939 ) ) ;
#4123=DIRECTION ( 'NONE',  ( 0.000000000000000000, 0.000000000000000000, -1.000000000000000000 ) ) ;
#4138=CARTESIAN_POINT ( 'NONE',  ( 33.00000000000000000, 0.000000000000000000, -41.99999999999999289 ) ) ;
#4147=VERTEX_POINT ( 'NONE', #4636 ) ;
#4160=ORIENTED_EDGE ( 'NONE', *, *, #12157, .T. ) ;
#4165=FACE_OUTER_BOUND ( 'NONE', #829, .T. ) ;
#4169=DIRECTION ( 'NONE',  ( -1.000000000000000000, -0.000000000000000000, -0.000000000000000000 ) ) ;
#4178=FACE_OUTER_BOUND ( 'NONE', #11138, .T. ) ;
#4184=CARTESIAN_POINT ( 'NONE',  ( 33.00000000000000000, 0.000000000000000000, -49.49999999999999289 ) ) ;
#4185=CARTESIAN_POINT ( 'NONE',  ( -36.00000000000000711, 34.64101615137755630, 20.00000000000001066 ) ) ;
#4189=ORIENTED_EDGE ( 'NONE', *, *, #3411, .T. ) ;
#4191=LINE ( 'NONE', #10887, #37 ) ;
#4203=LINE ( 'NONE', #1468, #2838 ) ;
#4205=DIRECTION ( 'NONE',  ( 0.000000000000000000, 0.000000000000000000, -1.000000000000000000 ) ) ;
#4209=ADVANCED_BREP_SHAPE_REPRESENTATION ( '', ( #313, #6056 ), #6251 ) ;
#4210=AXIS2_PLACEMENT_3D ( 'NONE', #11476, #2053, #2924 ) ;
#4216=AXIS2_PLACEMENT_3D ( 'NONE', #6617, #2675, #6262 ) ;
#4219=VECTOR ( 'NONE', #8044, 1000.000000000000000 ) ;
#4233=VECTOR ( 'NONE', #11938, 1000.000000000000000 ) ;
#4246=EDGE_CURVE ( 'NONE', #4605, #3761, #3671, .T. ) ;
#4253=CYLINDRICAL_SURFACE ( 'NONE', #9408, 1.999999999999998224 ) ;
#4276=CARTESIAN_POINT ( 'NONE',  ( -33.00000000000000000, 0.000000000000000000, -7.500000000000000888 ) ) ;
#4278=ORIENTED_EDGE ( 'NONE', *, *, #4901, .F. ) ;
#4294=LINE ( 'NONE', #11855, #6201 ) ;
#4316=ORIENTED_EDGE ( 'NONE', *, *, #6114, .T. ) ;
#4340=DIRECTION ( 'NONE',  ( 0.000000000000000000, 0.000000000000000000, -1.000000000000000000 ) ) ;
#4343=ORIENTED_EDGE ( 'NONE', *, *, #3578, .T. ) ;
#4348=DIRECTION ( 'NONE',  ( -1.000000000000000000, 0.000000000000000000, 0.000000000000000000 ) ) ;
#4353=AXIS2_PLACEMENT_3D ( 'NONE', #1938, #1806, #8441 ) ;
#4354=ORIENTED_EDGE ( 'NONE', *, *, #10735, .T. ) ;
#4359=ORIENTED_EDGE ( 'NONE', *, *, #2422, .T. ) ;
#4365=CARTESIAN_POINT ( 'NONE',  ( -15.00000000000000000, 40.00000000000000711, 2.000000000000000000 ) ) ;
#4415=LINE ( 'NONE', #2482, #12147 ) ;
#4418=CIRCLE ( 'NONE', #4210, 6.500000000000000888 ) ;
#4423=EDGE_CURVE ( 'NONE', #1692, #6339, #3278, .T. ) ;
#4427=ORIENTED_EDGE ( 'NONE', *, *, #4498, .F. ) ;
#4433=ORIENTED_EDGE ( 'NONE', *, *, #3578, .F. ) ;
#4434=CARTESIAN_POINT ( 'NONE',  ( 33.00000000000000000, 0.000000000000000000, 0.000000000000000000 ) ) ;
#4441=CARTESIAN_POINT ( 'NONE',  ( 36.00000000000000711, 0.000000000000000000, -41.99999999999999289 ) ) ;
#4462=DIRECTION ( 'NONE',  ( 0.000000000000000000, 0.000000000000000000, -1.000000000000000000 ) ) ;
#4471=EDGE_CURVE ( 'NONE', #6982, #1491, #2281, .T. ) ;
#4476=CARTESIAN_POINT ( 'NONE',  ( 28.99999999999999645, 0.000000000000000000, -41.99999999999999289 ) ) ;
#4495=CARTESIAN_POINT ( 'NONE',  ( 29.00000000000000000, 0.000000000000000000, -41.99999999999999289 ) ) ;
#4496=VERTEX_POINT ( 'NONE', #3969 ) ;
#4498=EDGE_CURVE ( 'NONE', #11527, #4496, #4783, .T. ) ;
#4499=EDGE_CURVE ( 'NONE', #4951, #3355, #10593, .T. ) ;
#4530=ORIENTED_EDGE ( 'NONE', *, *, #2803, .T. ) ;
#4588=STYLED_ITEM('',(#12377),#313);
#4590=CARTESIAN_POINT ( 'NONE',  ( 29.00000000000000000, 9.184850993605147944E-16, -49.49999999999999289 ) ) ;
#4605=VERTEX_POINT ( 'NONE', #1215 ) ;
#4622=CYLINDRICAL_SURFACE ( 'NONE', #4353, 5.199999999999996625 ) ;
#4627=CIRCLE ( 'NONE', #4216, 40.00000000000000711 ) ;
#4636=CARTESIAN_POINT ( 'NONE',  ( -36.00000000000000711, 0.000000000000000000, -7.500000000000000888 ) ) ;
#4638=CARTESIAN_POINT ( 'NONE',  ( 33.00000000000000000, 0.000000000000000000, -41.99999999999999289 ) ) ;
#4639=VERTEX_POINT ( 'NONE', #4276 ) ;
#4653=CIRCLE ( 'NONE', #6058, 6.500000000000000888 ) ;
#4663=CARTESIAN_POINT ( 'NONE',  ( -36.00000000000000711, 0.000000000000000000, 0.000000000000000000 ) ) ;
#4667=ORIENTED_EDGE ( 'NONE', *, *, #4471, .T. ) ;
#4673=LINE ( 'NONE', #9358, #10609 ) ;
#4674=DIRECTION ( 'NONE',  ( 0.000000000000000000, 0.000000000000000000, -1.000000000000000000 ) ) ;
#4678=CARTESIAN_POINT ( 'NONE',  ( 28.99999999999999645, 0.000000000000000000, -41.99999999999999289 ) ) ;
#4721=CARTESIAN_POINT ( 'NONE',  ( 15.00000000000000355, 40.00000000000000711, 0.000000000000000000 ) ) ;
#4723=DIRECTION ( 'NONE',  ( -0.000000000000000000, 1.000000000000000000, -0.000000000000000000 ) ) ;
#4736=CARTESIAN_POINT ( 'NONE',  ( -33.00000000000000000, 0.000000000000000000, 0.000000000000000000 ) ) ;
#4769=CARTESIAN_POINT ( 'NONE',  ( -26.00000000000000355, 0.000000000000000000, 6.500000000000000888 ) ) ;
#4772=AXIS2_PLACEMENT_3D ( 'NONE', #5284, #6877, #4205 ) ;
#4777=EDGE_LOOP ( 'NONE', ( #8731, #1721 ) ) ;
#4783=LINE ( 'NONE', #8672, #4075 ) ;
#4788=DIRECTION ( 'NONE',  ( -1.000000000000000000, -0.000000000000000000, -0.000000000000000000 ) ) ;
#4795=DIRECTION ( 'NONE',  ( -0.000000000000000000, 1.000000000000000000, -0.000000000000000000 ) ) ;
#4801=ORIENTED_EDGE ( 'NONE', *, *, #12102, .T. ) ;
#4803=ORIENTED_EDGE ( 'NONE', *, *, #7002, .F. ) ;
#4823=AXIS2_PLACEMENT_3D ( 'NONE', #9, #9586, #9660 ) ;
#4824=AXIS2_PLACEMENT_3D ( 'NONE', #6789, #5663, #2033 ) ;
#4829=DIRECTION ( 'NONE',  ( 0.000000000000000000, -1.000000000000000000, 0.000000000000000000 ) ) ;
#4836=CARTESIAN_POINT ( 'NONE',  ( -36.00100000000000477, 6.368163355566235395E-16, -36.79999999999999716 ) ) ;
#4849=ORIENTED_EDGE ( 'NONE', *, *, #447, .T. ) ;
#4850=ORIENTED_EDGE ( 'NONE', *, *, #10117, .T. ) ;
#4855=VECTOR ( 'NONE', #6842, 1000.000000000000000 ) ;
#4860=EDGE_CURVE ( 'NONE', #2662, #1975, #10872, .T. ) ;
#4901=EDGE_CURVE ( 'NONE', #2661, #11627, #11510, .T. ) ;
#4907=ORIENTED_EDGE ( 'NONE', *, *, #7563, .T. ) ;
#4937=DIRECTION ( 'NONE',  ( 0.000000000000000000, 0.000000000000000000, 1.000000000000000000 ) ) ;
#4939=ADVANCED_FACE ( 'NONE', ( #8960 ), #203, .F. ) ;
#4941=VERTEX_POINT ( 'NONE', #3331 ) ;
#4944=CARTESIAN_POINT ( 'NONE',  ( 29.00000000000000000, 0.000000000000000000, -41.99999999999999289 ) ) ;
#4945=EDGE_CURVE ( 'NONE', #3376, #5880, #1288, .T. ) ;
#4949=CARTESIAN_POINT ( 'NONE',  ( 28.99999999999999645, 0.000000000000000000, -47.19999999999998863 ) ) ;
#4951=VERTEX_POINT ( 'NONE', #8846 ) ;
#4952=PLANE ( 'NONE',  #3686 ) ;
#4953=ORIENTED_EDGE ( 'NONE', *, *, #2422, .F. ) ;
#4963=AXIS2_PLACEMENT_3D ( 'NONE', #4663, #903, #8480 ) ;
#4968=AXIS2_PLACEMENT_3D ( 'NONE', #598, #10114, #5492 ) ;
#4978=CIRCLE ( 'NONE', #7182, 6.500000000000000888 ) ;
#5015=CARTESIAN_POINT ( 'NONE',  ( 33.00000000000000000, 0.000000000000000000, -41.99999999999999289 ) ) ;
#5027=CIRCLE ( 'NONE', #1637, 7.500000000000000888 ) ;
#5028=CIRCLE ( 'NONE', #9426, 40.00000000000000711 ) ;
#5037=ADVANCED_FACE ( 'NONE', ( #11697, #7090 ), #4952, .T. ) ;
#5048=PLANE ( 'NONE',  #11595 ) ;
#5061=ORIENTED_EDGE ( 'NONE', *, *, #5701, .T. ) ;
#5066=CARTESIAN_POINT ( 'NONE',  ( 36.00000000000000711, 34.64101615137755630, 20.00000000000001066 ) ) ;
#5110=EDGE_LOOP ( 'NONE', ( #9545, #11524, #5350, #3131 ) ) ;
#5128=PLANE ( 'NONE',  #3455 ) ;
#5129=LINE ( 'NONE', #3325, #9047 ) ;
#5135=DIRECTION ( 'NONE',  ( 1.000000000000000000, -0.000000000000000000, -0.000000000000000000 ) ) ;
#5146=CARTESIAN_POINT ( 'NONE',  ( -26.00000000000000355, 0.000000000000000000, 0.000000000000000000 ) ) ;
#5168=CARTESIAN_POINT ( 'NONE',  ( 36.00000000000000000, 30.00000000000000711, -19.99999999999998934 ) ) ;
#5172=CIRCLE ( 'NONE', #572, 7.500000000000000000 ) ;
#5196=EDGE_LOOP ( 'NONE', ( #9540, #5379, #2688, #7059 ) ) ;
#5204=CYLINDRICAL_SURFACE ( 'NONE', #10833, 1.999999999999998224 ) ;
#5230=VERTEX_POINT ( 'NONE', #12000 ) ;
#5238=ADVANCED_FACE ( 'NONE', ( #6759 ), #2941, .F. ) ;
#5242=EDGE_LOOP ( 'NONE', ( #3275, #8405, #11043, #5061, #4850, #322 ) ) ;
#5250=ORIENTED_EDGE ( 'NONE', *, *, #2581, .F. ) ;
#5257=CIRCLE ( 'NONE', #5862, 40.00000000000000711 ) ;
#5270=DIRECTION ( 'NONE',  ( 0.000000000000000000, 0.000000000000000000, -1.000000000000000000 ) ) ;
#5271=EDGE_CURVE ( 'NONE', #6734, #2662, #1096, .T. ) ;
#5284=CARTESIAN_POINT ( 'NONE',  ( -33.00000000000000000, 0.000000000000000000, 0.000000000000000000 ) ) ;
#5308=ORIENTED_EDGE ( 'NONE', *, *, #3163, .T. ) ;
#5315=EDGE_CURVE ( 'NONE', #451, #11627, #10685, .T. ) ;
#5325=CARTESIAN_POINT ( 'NONE',  ( -15.00000000000000000, 30.00000000000000711, -2.000000000000000000 ) ) ;
#5339=CARTESIAN_POINT ( 'NONE',  ( -26.00000000000000355, 30.00000000000000711, 20.00000000000001066 ) ) ;
#5350=ORIENTED_EDGE ( 'NONE', *, *, #7079, .T. ) ;
#5351=DIRECTION ( 'NONE',  ( 0.000000000000000000, 0.000000000000000000, 1.000000000000000000 ) ) ;
#5357=DIRECTION ( 'NONE',  ( -0.000000000000000000, -0.000000000000000000, 1.000000000000000000 ) ) ;
#5372=AXIS2_PLACEMENT_3D ( 'NONE', #7344, #8284, #6340 ) ;
#5379=ORIENTED_EDGE ( 'NONE', *, *, #567, .T. ) ;
#5390=ADVANCED_FACE ( 'NONE', ( #4178 ), #6896, .T. ) ;
#5394=FACE_OUTER_BOUND ( 'NONE', #7682, .T. ) ;
#5395=MECHANICAL_DESIGN_GEOMETRIC_PRESENTATION_REPRESENTATION('',(#4588),#3210);
#5412=DIRECTION ( 'NONE',  ( 0.000000000000000000, 0.000000000000000000, 1.000000000000000000 ) ) ;
#5417=CIRCLE ( 'NONE', #1825, 7.500000000000000000 ) ;
#5447=CARTESIAN_POINT ( 'NONE',  ( 36.00000000000000000, 30.00000000000000711, -19.99999999999998934 ) ) ;
#5452=SHAPE_REPRESENTATION_RELATIONSHIP ( 'NONE' , 'NONE' ,  #8907, #4209 ) ;
#5454=AXIS2_PLACEMENT_3D ( 'NONE', #3507, #3691, #688 ) ;
#5463=EDGE_CURVE ( 'NONE', #2486, #5230, #9098, .T. ) ;
#5466=DIRECTION ( 'NONE',  ( 0.000000000000000000, 0.000000000000000000, 1.000000000000000000 ) ) ;
#5474=AXIS2_PLACEMENT_3D ( 'NONE', #591, #2722, #6539 ) ;
#5480=CARTESIAN_POINT ( 'NONE',  ( 36.00000000000000711, 7.960204194457796463E-16, -6.500000000000000888 ) ) ;
#5481=ORIENTED_EDGE ( 'NONE', *, *, #6717, .T. ) ;
#5482=EDGE_CURVE ( 'NONE', #9771, #3971, #4069, .T. ) ;
#5490=ORIENTED_EDGE ( 'NONE', *, *, #2581, .T. ) ;
#5492=DIRECTION ( 'NONE',  ( 0.000000000000000000, 0.000000000000000000, -1.000000000000000000 ) ) ;
#5519=DIRECTION ( 'NONE',  ( -0.000000000000000000, 1.000000000000000000, -0.000000000000000000 ) ) ;
#5525=EDGE_LOOP ( 'NONE', ( #532, #4433, #755, #4359 ) ) ;
#5526=EDGE_CURVE ( 'NONE', #7918, #451, #7320, .T. ) ;
#5531=CYLINDRICAL_SURFACE ( 'NONE', #2834, 6.500000000000000888 ) ;
#5542=CARTESIAN_POINT ( 'NONE',  ( -36.00000000000000000, 30.00000000000000711, 20.00000000000001066 ) ) ;
#5545=ORIENTED_EDGE ( 'NONE', *, *, #10306, .F. ) ;
#5567=ADVANCED_FACE ( 'NONE', ( #11059 ), #2429, .F. ) ;
#5568=AXIS2_PLACEMENT_3D ( 'NONE', #10096, #12015, #4462 ) ;
#5577=ORIENTED_EDGE ( 'NONE', *, *, #6629, .F. ) ;
#5581=VERTEX_POINT ( 'NONE', #682 ) ;
#5589=CARTESIAN_POINT ( 'NONE',  ( 33.00000000000000000, 9.184850993605149917E-16, 7.500000000000000888 ) ) ;
#5600=FACE_OUTER_BOUND ( 'NONE', #11806, .T. ) ;
#5609=ORIENTED_EDGE ( 'NONE', *, *, #7312, .F. ) ;
#5625=DIRECTION ( 'NONE',  ( 0.000000000000000000, 0.000000000000000000, 1.000000000000000000 ) ) ;
#5628=ORIENTED_EDGE ( 'NONE', *, *, #7693, .F. ) ;
#5639=VECTOR ( 'NONE', #7944, 1000.000000000000000 ) ;
#5644=EDGE_LOOP ( 'NONE', ( #5609, #298, #264, #6578 ) ) ;
#5663=DIRECTION ( 'NONE',  ( 1.000000000000000000, -0.000000000000000000, -0.000000000000000000 ) ) ;
#5681=ORIENTED_EDGE ( 'NONE', *, *, #11489, .F. ) ;
#5690=AXIS2_PLACEMENT_3D ( 'NONE', #7894, #8006, #11626 ) ;
#5691=DIRECTION ( 'NONE',  ( 1.000000000000000000, 0.000000000000000000, 0.000000000000000000 ) ) ;
#5697=DIRECTION ( 'NONE',  ( 0.000000000000000000, 0.000000000000000000, 1.000000000000000000 ) ) ;
#5698=ORIENTED_EDGE ( 'NONE', *, *, #4499, .F. ) ;
#5701=EDGE_CURVE ( 'NONE', #11004, #5845, #6503, .T. ) ;
#5712=ORIENTED_EDGE ( 'NONE', *, *, #3192, .T. ) ;
#5731=DIRECTION ( 'NONE',  ( 0.000000000000000000, 0.000000000000000000, -1.000000000000000000 ) ) ;
#5749=CARTESIAN_POINT ( 'NONE',  ( 36.00000000000000711, 0.000000000000000000, 0.000000000000000000 ) ) ;
#5753=AXIS2_PLACEMENT_3D ( 'NONE', #4434, #6317, #11244 ) ;
#5767=CIRCLE ( 'NONE', #9168, 1.999999999999998224 ) ;
#5779=DIRECTION ( 'NONE',  ( -1.000000000000000000, 0.000000000000000000, 0.000000000000000000 ) ) ;
#5798=DIRECTION ( 'NONE',  ( 0.000000000000000000, 0.000000000000000000, 1.000000000000000000 ) ) ;
#5805=ORIENTED_EDGE ( 'NONE', *, *, #9133, .T. ) ;
#5808=ORIENTED_EDGE ( 'NONE', *, *, #11489, .T. ) ;
#5817=EDGE_LOOP ( 'NONE', ( #4907, #9142 ) ) ;
#5825=ORIENTED_EDGE ( 'NONE', *, *, #8386, .F. ) ;
#5830=CIRCLE ( 'NONE', #426, 7.500000000000000000 ) ;
#5834=CARTESIAN_POINT ( 'NONE',  ( -36.00000000000000000, 40.00000000000000711, 20.00000000000001066 ) ) ;
#5845=VERTEX_POINT ( 'NONE', #7747 ) ;
#5862=AXIS2_PLACEMENT_3D ( 'NONE', #8953, #8901, #315 ) ;
#5863=AXIS2_PLACEMENT_3D ( 'NONE', #3328, #7140, #8382 ) ;
#5873=CARTESIAN_POINT ( 'NONE',  ( 36.00000000000000711, 0.000000000000000000, 0.000000000000000000 ) ) ;
#5876=AXIS2_PLACEMENT_3D ( 'NONE', #2939, #9329, #4123 ) ;
#5880=VERTEX_POINT ( 'NONE', #115 ) ;
#5890=ORIENTED_EDGE ( 'NONE', *, *, #5701, .F. ) ;
#5900=CARTESIAN_POINT ( 'NONE',  ( 36.00000000000000711, 12.50000000000000000, -24.50000000000000000 ) ) ;
#5926=DIRECTION ( 'NONE',  ( 0.000000000000000000, 0.000000000000000000, -1.000000000000000000 ) ) ;
#5929=VERTEX_POINT ( 'NONE', #5933 ) ;
#5933=CARTESIAN_POINT ( 'NONE',  ( 36.00000000000000000, 34.64101615137755630, 20.00000000000001066 ) ) ;
#5938=CYLINDRICAL_SURFACE ( 'NONE', #6807, 40.00000000000000711 ) ;
#5955=FACE_OUTER_BOUND ( 'NONE', #8095, .T. ) ;
#5980=DIRECTION ( 'NONE',  ( -1.000000000000000000, -0.000000000000000000, -0.000000000000000000 ) ) ;
#5992=DIRECTION ( 'NONE',  ( 1.000000000000000000, 0.000000000000000000, 0.000000000000000000 ) ) ;
#5997=CARTESIAN_POINT ( 'NONE',  ( 36.00000000000000000, 40.00000000000000711, -19.99999999999998934 ) ) ;
#6023=DIRECTION ( 'NONE',  ( -1.000000000000000000, -0.000000000000000000, -0.000000000000000000 ) ) ;
#6032=AXIS2_PLACEMENT_3D ( 'NONE', #3120, #4795, #5798 ) ;
#6051=DIRECTION ( 'NONE',  ( -1.000000000000000000, 0.000000000000000000, 0.000000000000000000 ) ) ;
#6056=AXIS2_PLACEMENT_3D ( 'NONE', #212, #4035, #8864 ) ;
#6058=AXIS2_PLACEMENT_3D ( 'NONE', #11993, #2551, #8270 ) ;
#6075=EDGE_CURVE ( 'NONE', #4941, #6339, #12092, .T. ) ;
#6084=DIRECTION ( 'NONE',  ( -1.000000000000000000, -0.000000000000000000, -0.000000000000000000 ) ) ;
#6096=CARTESIAN_POINT ( 'NONE',  ( -33.00000000000000000, 0.000000000000000000, 0.000000000000000000 ) ) ;
#6112=DIRECTION ( 'NONE',  ( 1.000000000000000000, 0.000000000000000000, 0.000000000000000000 ) ) ;
#6114=EDGE_CURVE ( 'NONE', #4049, #2452, #4673, .T. ) ;
#6117=CARTESIAN_POINT ( 'NONE',  ( 33.00000000000000000, 9.184850993605147944E-16, -34.49999999999999289 ) ) ;
#6122=ORIENTED_EDGE ( 'NONE', *, *, #5463, .F. ) ;
#6127=PRODUCT ( 'main body', 'main body', '', ( #100 ) ) ;
#6129=CARTESIAN_POINT ( 'NONE',  ( 36.00000000000000711, -12.50000000000000000, -37.99671038392666134 ) ) ;
#6141=ORIENTED_EDGE ( 'NONE', *, *, #6075, .F. ) ;
#6146=DIRECTION ( 'NONE',  ( -0.000000000000000000, 1.000000000000000000, -0.000000000000000000 ) ) ;
#6156=AXIS2_PLACEMENT_3D ( 'NONE', #12235, #10550, #6699 ) ;
#6170=CIRCLE ( 'NONE', #5372, 7.500000000000000888 ) ;
#6201=VECTOR ( 'NONE', #4169, 1000.000000000000000 ) ;
#6212=DIRECTION ( 'NONE',  ( 0.000000000000000000, 0.000000000000000000, -1.000000000000000000 ) ) ;
#6230=AXIS2_PLACEMENT_3D ( 'NONE', #6096, #3288, #6212 ) ;
#6246=ADVANCED_FACE ( 'NONE', ( #9097 ), #10942, .F. ) ;
#6251=( GEOMETRIC_REPRESENTATION_CONTEXT ( 3 ) GLOBAL_UNCERTAINTY_ASSIGNED_CONTEXT ( ( #11511 ) ) GLOBAL_UNIT_ASSIGNED_CONTEXT ( ( #2556, #6270, #2625 ) ) REPRESENTATION_CONTEXT ( 'NONE', 'WORKASPACE' ) );
#6257=DIRECTION ( 'NONE',  ( 1.000000000000000000, -0.000000000000000000, -0.000000000000000000 ) ) ;
#6260=AXIS2_PLACEMENT_3D ( 'NONE', #11923, #7332, #10187 ) ;
#6262=DIRECTION ( 'NONE',  ( 0.000000000000000000, 0.000000000000000000, -1.000000000000000000 ) ) ;
#6270=( NAMED_UNIT ( * ) PLANE_ANGLE_UNIT ( ) SI_UNIT ( $, .RADIAN. ) );
#6293=CARTESIAN_POINT ( 'NONE',  ( -13.05124837953327344, 0.000000000000000000, -54.50000000000000000 ) ) ;
#6296=DIRECTION ( 'NONE',  ( 0.000000000000000000, 0.000000000000000000, -1.000000000000000000 ) ) ;
#6299=ORIENTED_EDGE ( 'NONE', *, *, #2432, .F. ) ;
#6310=ORIENTED_EDGE ( 'NONE', *, *, #8084, .F. ) ;
#6316=EDGE_LOOP ( 'NONE', ( #11077, #844, #5805, #10213, #8098, #9589, #1697, #11203 ) ) ;
#6317=DIRECTION ( 'NONE',  ( 1.000000000000000000, 0.000000000000000000, 0.000000000000000000 ) ) ;
#6326=FILL_AREA_STYLE_COLOUR ( '', #1427 ) ;
#6338=LINE ( 'NONE', #8155, #4233 ) ;
#6339=VERTEX_POINT ( 'NONE', #3334 ) ;
#6340=DIRECTION ( 'NONE',  ( 0.000000000000000000, 0.000000000000000000, -1.000000000000000000 ) ) ;
#6355=ORIENTED_EDGE ( 'NONE', *, *, #5482, .F. ) ;
#6357=FACE_OUTER_BOUND ( 'NONE', #11602, .T. ) ;
#6369=VECTOR ( 'NONE', #4348, 1000.000000000000000 ) ;
#6375=DIRECTION ( 'NONE',  ( -1.000000000000000000, -0.000000000000000000, -0.000000000000000000 ) ) ;
#6376=DIRECTION ( 'NONE',  ( 0.000000000000000000, -0.000000000000000000, -1.000000000000000000 ) ) ;
#6380=( NAMED_UNIT ( * ) SI_UNIT ( $, .STERADIAN. ) SOLID_ANGLE_UNIT ( ) );
#6385=VECTOR ( 'NONE', #3945, 1000.000000000000000 ) ;
#6395=DIRECTION ( 'NONE',  ( 0.000000000000000000, 0.000000000000000000, 1.000000000000000000 ) ) ;
#6454=( LENGTH_UNIT ( ) NAMED_UNIT ( * ) SI_UNIT ( .MILLI., .METRE. ) );
#6487=ORIENTED_EDGE ( 'NONE', *, *, #4423, .T. ) ;
#6492=PLANE ( 'NONE',  #3183 ) ;
#6493=AXIS2_PLACEMENT_3D ( 'NONE', #5749, #7457, #5697 ) ;
#6503=LINE ( 'NONE', #12294, #12074 ) ;
#6518=CARTESIAN_POINT ( 'NONE',  ( 36.00000000000000000, 40.00000000000000711, 20.00000000000001066 ) ) ;
#6531=LINE ( 'NONE', #9167, #12185 ) ;
#6533=FACE_OUTER_BOUND ( 'NONE', #10177, .T. ) ;
#6539=DIRECTION ( 'NONE',  ( 0.000000000000000000, 0.000000000000000000, -1.000000000000000000 ) ) ;
#6552=CARTESIAN_POINT ( 'NONE',  ( 36.00000000000000711, 0.000000000000000000, 0.000000000000000000 ) ) ;
#6559=DIRECTION ( 'NONE',  ( 1.000000000000000000, 0.000000000000000000, 0.000000000000000000 ) ) ;
#6562=CIRCLE ( 'NONE', #4963, 40.00000000000000711 ) ;
#6571=EDGE_LOOP ( 'NONE', ( #12196, #10172 ) ) ;
#6574=CIRCLE ( 'NONE', #10766, 40.00000000000000711 ) ;
#6578=ORIENTED_EDGE ( 'NONE', *, *, #7079, .F. ) ;
#6583=EDGE_LOOP ( 'NONE', ( #3302, #2159 ) ) ;
#6584=DIRECTION ( 'NONE',  ( -0.000000000000000000, 1.000000000000000000, -0.000000000000000000 ) ) ;
#6585=DIRECTION ( 'NONE',  ( 0.000000000000000000, 0.000000000000000000, -1.000000000000000000 ) ) ;
#6588=DIRECTION ( 'NONE',  ( -1.000000000000000000, -0.000000000000000000, -0.000000000000000000 ) ) ;
#6594=CARTESIAN_POINT ( 'NONE',  ( -36.00000000000000711, 0.000000000000000000, 40.00000000000000711 ) ) ;
#6597=VERTEX_POINT ( 'NONE', #7516 ) ;
#6602=CARTESIAN_POINT ( 'NONE',  ( 15.00000000000000355, 40.00000000000000711, 0.000000000000000000 ) ) ;
#6612=CIRCLE ( 'NONE', #8820, 5.199999999999996625 ) ;
#6617=CARTESIAN_POINT ( 'NONE',  ( 26.00000000000000355, 0.000000000000000000, 0.000000000000000000 ) ) ;
#6624=AXIS2_PLACEMENT_3D ( 'NONE', #4476, #3725, #8298 ) ;
#6629=EDGE_CURVE ( 'NONE', #1320, #1424, #8518, .T. ) ;
#6636=LINE ( 'NONE', #3882, #4002 ) ;
#6642=DIRECTION ( 'NONE',  ( 0.000000000000000000, 0.000000000000000000, -1.000000000000000000 ) ) ;
#6659=ORIENTED_EDGE ( 'NONE', *, *, #9595, .F. ) ;
#6660=DIRECTION ( 'NONE',  ( -1.000000000000000000, -0.000000000000000000, -0.000000000000000000 ) ) ;
#6690=DIRECTION ( 'NONE',  ( 1.000000000000000000, -0.000000000000000000, -0.000000000000000000 ) ) ;
#6699=DIRECTION ( 'NONE',  ( 0.000000000000000000, 0.000000000000000000, -1.000000000000000000 ) ) ;
#6702=EDGE_CURVE ( 'NONE', #2147, #11069, #3085, .T. ) ;
#6707=EDGE_LOOP ( 'NONE', ( #11890, #8973, #2463, #5808 ) ) ;
#6709=DIRECTION ( 'NONE',  ( 0.000000000000000000, 0.000000000000000000, -1.000000000000000000 ) ) ;
#6717=EDGE_CURVE ( 'NONE', #10764, #1709, #1363, .T. ) ;
#6734=VERTEX_POINT ( 'NONE', #2362 ) ;
#6747=DIRECTION ( 'NONE',  ( 0.000000000000000000, 0.000000000000000000, -1.000000000000000000 ) ) ;
#6759=FACE_OUTER_BOUND ( 'NONE', #8669, .T. ) ;
#6764=AXIS2_PLACEMENT_3D ( 'NONE', #726, #7179, #10167 ) ;
#6769=PLANE ( 'NONE',  #1639 ) ;
#6773=CIRCLE ( 'NONE', #4968, 7.500000000000000888 ) ;
#6780=ADVANCED_FACE ( 'NONE', ( #4072 ), #7007, .T. ) ;
#6785=DIRECTION ( 'NONE',  ( -1.000000000000000000, 0.000000000000000000, 0.000000000000000000 ) ) ;
#6789=CARTESIAN_POINT ( 'NONE',  ( -36.00000000000000711, 0.000000000000000000, 0.000000000000000000 ) ) ;
#6791=ORIENTED_EDGE ( 'NONE', *, *, #11883, .T. ) ;
#6796=AXIS2_PLACEMENT_3D ( 'NONE', #11267, #6584, #2900 ) ;
#6807=AXIS2_PLACEMENT_3D ( 'NONE', #1878, #11614, #1065 ) ;
#6811=EDGE_CURVE ( 'NONE', #8658, #7148, #2386, .T. ) ;
#6816=DIRECTION ( 'NONE',  ( 0.000000000000000000, 0.000000000000000000, 1.000000000000000000 ) ) ;
#6842=DIRECTION ( 'NONE',  ( 0.000000000000000000, 1.000000000000000000, 0.000000000000000000 ) ) ;
#6862=VERTEX_POINT ( 'NONE', #10004 ) ;
#6877=DIRECTION ( 'NONE',  ( 1.000000000000000000, -0.000000000000000000, -0.000000000000000000 ) ) ;
#6896=CYLINDRICAL_SURFACE ( 'NONE', #5690, 40.00000000000000711 ) ;
#6906=DIRECTION ( 'NONE',  ( 0.000000000000000000, 0.000000000000000000, 1.000000000000000000 ) ) ;
#6914=DIRECTION ( 'NONE',  ( 0.000000000000000000, 0.000000000000000000, -1.000000000000000000 ) ) ;
#6920=ORIENTED_EDGE ( 'NONE', *, *, #8854, .F. ) ;
#6924=ORIENTED_EDGE ( 'NONE', *, *, #12157, .F. ) ;
#6949=DIRECTION ( 'NONE',  ( 1.000000000000000000, -0.000000000000000000, -0.000000000000000000 ) ) ;
#6960=ORIENTED_EDGE ( 'NONE', *, *, #6717, .F. ) ;
#6974=AXIS2_PLACEMENT_3D ( 'NONE', #4736, #2056, #6747 ) ;
#6976=ORIENTED_EDGE ( 'NONE', *, *, #807, .F. ) ;
#6979=LINE ( 'NONE', #7875, #7627 ) ;
#6982=VERTEX_POINT ( 'NONE', #2877 ) ;
#6985=VECTOR ( 'NONE', #7831, 1000.000000000000000 ) ;
#7002=EDGE_CURVE ( 'NONE', #2114, #1494, #9765, .T. ) ;
#7007=CYLINDRICAL_SURFACE ( 'NONE', #8787, 40.00000000000000711 ) ;
#7017=CARTESIAN_POINT ( 'NONE',  ( -26.00000000000000355, 0.000000000000000000, 40.00000000000000711 ) ) ;
#7049=EDGE_LOOP ( 'NONE', ( #9995, #3564, #7189, #4667 ) ) ;
#7055=DIRECTION ( 'NONE',  ( -0.000000000000000000, 1.000000000000000000, -0.000000000000000000 ) ) ;
#7059=ORIENTED_EDGE ( 'NONE', *, *, #1742, .F. ) ;
#7079=EDGE_CURVE ( 'NONE', #8658, #2298, #10433, .T. ) ;
#7082=AXIS2_PLACEMENT_3D ( 'NONE', #6602, #4723, #964 ) ;
#7090=FACE_BOUND ( 'NONE', #8517, .T. ) ;
#7091=ORIENTED_EDGE ( 'NONE', *, *, #11134, .T. ) ;
#7094=ADVANCED_FACE ( 'NONE', ( #794 ), #4622, .F. ) ;
#7115=CARTESIAN_POINT ( 'NONE',  ( -15.00000000000000000, 30.00000000000000711, 0.000000000000000000 ) ) ;
#7126=ORIENTED_EDGE ( 'NONE', *, *, #3099, .F. ) ;
#7128=DIRECTION ( 'NONE',  ( 0.000000000000000000, 0.000000000000000000, 1.000000000000000000 ) ) ;
#7140=DIRECTION ( 'NONE',  ( -0.000000000000000000, 1.000000000000000000, 0.000000000000000000 ) ) ;
#7147=CARTESIAN_POINT ( 'NONE',  ( -15.00000000000000000, 40.00000000000000711, 0.000000000000000000 ) ) ;
#7148=VERTEX_POINT ( 'NONE', #1299 ) ;
#7179=DIRECTION ( 'NONE',  ( 1.000000000000000000, 0.000000000000000000, 0.000000000000000000 ) ) ;
#7182=AXIS2_PLACEMENT_3D ( 'NONE', #1156, #8800, #5731 ) ;
#7186=ADVANCED_FACE ( 'NONE', ( #4165 ), #9749, .F. ) ;
#7189=ORIENTED_EDGE ( 'NONE', *, *, #8386, .T. ) ;
#7195=CARTESIAN_POINT ( 'NONE',  ( -33.00000000000000000, 0.000000000000000000, 0.000000000000000000 ) ) ;
#7206=ORIENTED_EDGE ( 'NONE', *, *, #8716, .T. ) ;
#7211=CIRCLE ( 'NONE', #2015, 7.500000000000000000 ) ;
#7222=DIRECTION ( 'NONE',  ( 1.000000000000000000, -0.000000000000000000, -0.000000000000000000 ) ) ;
#7254=DIRECTION ( 'NONE',  ( 0.000000000000000000, 0.000000000000000000, -1.000000000000000000 ) ) ;
#7267=EDGE_CURVE ( 'NONE', #8289, #3971, #3176, .T. ) ;
#7269=ADVANCED_FACE ( 'NONE', ( #6357 ), #10235, .T. ) ;
#7273=DIRECTION ( 'NONE',  ( 1.000000000000000000, -0.000000000000000000, -0.000000000000000000 ) ) ;
#7287=PLANE ( 'NONE',  #3062 ) ;
#7300=VECTOR ( 'NONE', #11805, 1000.000000000000000 ) ;
#7312=EDGE_CURVE ( 'NONE', #7148, #8658, #6773, .T. ) ;
#7320=LINE ( 'NONE', #1684, #10097 ) ;
#7322=EDGE_CURVE ( 'NONE', #10639, #1934, #4415, .T. ) ;
#7328=CARTESIAN_POINT ( 'NONE',  ( 33.00000000000000000, 0.000000000000000000, 0.000000000000000000 ) ) ;
#7329=FACE_OUTER_BOUND ( 'NONE', #6707, .T. ) ;
#7332=DIRECTION ( 'NONE',  ( -1.000000000000000000, 0.000000000000000000, 0.000000000000000000 ) ) ;
#7341=DIRECTION ( 'NONE',  ( -0.000000000000000000, 1.000000000000000000, 0.000000000000000000 ) ) ;
#7344=CARTESIAN_POINT ( 'NONE',  ( -36.00000000000000711, 0.000000000000000000, 0.000000000000000000 ) ) ;
#7346=CARTESIAN_POINT ( 'NONE',  ( 26.00000000000000355, 0.000000000000000000, -19.99999999999998934 ) ) ;
#7383=CARTESIAN_POINT ( 'NONE',  ( 36.00000000000000000, 40.00000000000000711, 20.00000000000001066 ) ) ;
#7384=EDGE_CURVE ( 'NONE', #231, #3450, #1489, .T. ) ;
#7399=CIRCLE ( 'NONE', #603, 6.500000000000000888 ) ;
#7400=FACE_BOUND ( 'NONE', #2764, .T. ) ;
#7410=ADVANCED_FACE ( 'NONE', ( #1790, #5600, #1925 ), #6492, .F. ) ;
#7420=CIRCLE ( 'NONE', #6032, 2.000000000000000000 ) ;
#7444=EDGE_CURVE ( 'NONE', #9986, #2114, #3789, .T. ) ;
#7457=DIRECTION ( 'NONE',  ( -1.000000000000000000, -0.000000000000000000, -0.000000000000000000 ) ) ;
#7463=ADVANCED_FACE ( 'NONE', ( #780 ), #11289, .F. ) ;
#7496=ORIENTED_EDGE ( 'NONE', *, *, #11192, .T. ) ;
#7501=ORIENTED_EDGE ( 'NONE', *, *, #7384, .T. ) ;
#7508=DIRECTION ( 'NONE',  ( 0.000000000000000000, 0.000000000000000000, -1.000000000000000000 ) ) ;
#7516=CARTESIAN_POINT ( 'NONE',  ( 15.00000000000000355, 30.00000000000000711, 1.999999999999998224 ) ) ;
#7530=( NAMED_UNIT ( * ) SI_UNIT ( $, .STERADIAN. ) SOLID_ANGLE_UNIT ( ) );
#7541=ADVANCED_FACE ( 'NONE', ( #10954 ), #2392, .F. ) ;
#7563=EDGE_CURVE ( 'NONE', #4147, #3450, #6170, .T. ) ;
#7596=CARTESIAN_POINT ( 'NONE',  ( -36.00000000000000711, 0.000000000000000000, 0.000000000000000000 ) ) ;
#7598=ORIENTED_EDGE ( 'NONE', *, *, #1317, .F. ) ;
#7600=DIRECTION ( 'NONE',  ( 0.000000000000000000, 0.000000000000000000, 1.000000000000000000 ) ) ;
#7627=VECTOR ( 'NONE', #3978, 1000.000000000000000 ) ;
#7633=EDGE_CURVE ( 'NONE', #2426, #6734, #11024, .T. ) ;
#7635=DIRECTION ( 'NONE',  ( 1.000000000000000000, -0.000000000000000000, -0.000000000000000000 ) ) ;
#7655=DIRECTION ( 'NONE',  ( -0.000000000000000000, -0.000000000000000000, 1.000000000000000000 ) ) ;
#7675=ORIENTED_EDGE ( 'NONE', *, *, #9074, .F. ) ;
#7682=EDGE_LOOP ( 'NONE', ( #1813, #2394, #4801, #3891 ) ) ;
#7693=EDGE_CURVE ( 'NONE', #10319, #2452, #3982, .T. ) ;
#7698=CARTESIAN_POINT ( 'NONE',  ( 33.00000000000000000, 0.000000000000000000, -7.500000000000000888 ) ) ;
#7708=CARTESIAN_POINT ( 'NONE',  ( -15.00000000000000000, 30.00000000000000711, 2.000000000000000000 ) ) ;
#7711=DIRECTION ( 'NONE',  ( 0.000000000000000000, 0.000000000000000000, -1.000000000000000000 ) ) ;
#7718=ORIENTED_EDGE ( 'NONE', *, *, #7633, .T. ) ;
#7725=CARTESIAN_POINT ( 'NONE',  ( 15.00000000000000355, 40.00000000000000711, -1.999999999999998224 ) ) ;
#7735=SHAPE_DEFINITION_REPRESENTATION ( #10818, #8907 ) ;
#7747=CARTESIAN_POINT ( 'NONE',  ( -26.00000000000000355, 30.00000000000000711, -19.99999999999998934 ) ) ;
#7754=FACE_OUTER_BOUND ( 'NONE', #5242, .T. ) ;
#7772=FACE_OUTER_BOUND ( 'NONE', #9125, .T. ) ;
#7779=ORIENTED_EDGE ( 'NONE', *, *, #10305, .T. ) ;
#7792=UNCERTAINTY_MEASURE_WITH_UNIT (LENGTH_MEASURE( 1.000000000000000082E-05 ), #10329, 'distance_accuracy_value', 'NONE');
#7794=AXIS2_PLACEMENT_3D ( 'NONE', #8680, #10673, #10855 ) ;
#7831=DIRECTION ( 'NONE',  ( -1.000000000000000000, -0.000000000000000000, -0.000000000000000000 ) ) ;
#7839=CARTESIAN_POINT ( 'NONE',  ( 26.00000000000000355, -12.50000000000000000, -24.50000000000000000 ) ) ;
#7845=FACE_OUTER_BOUND ( 'NONE', #1874, .T. ) ;
#7862=DIRECTION ( 'NONE',  ( 0.000000000000000000, 0.000000000000000000, 1.000000000000000000 ) ) ;
#7867=ADVANCED_FACE ( 'NONE', ( #5955 ), #10759, .T. ) ;
#7875=CARTESIAN_POINT ( 'NONE',  ( 26.00000000000000355, 0.000000000000000000, 20.00000000000001066 ) ) ;
#7894=CARTESIAN_POINT ( 'NONE',  ( 36.00000000000000711, 0.000000000000000000, 0.000000000000000000 ) ) ;
#7901=DIRECTION ( 'NONE',  ( 0.000000000000000000, -0.000000000000000000, 1.000000000000000000 ) ) ;
#7918=VERTEX_POINT ( 'NONE', #4949 ) ;
#7929=CARTESIAN_POINT ( 'NONE',  ( 36.00000000000000711, 0.000000000000000000, -41.99999999999999289 ) ) ;
#7936=CARTESIAN_POINT ( 'NONE',  ( 33.00000000000000000, 0.000000000000000000, 0.000000000000000000 ) ) ;
#7944=DIRECTION ( 'NONE',  ( 1.000000000000000000, -0.000000000000000000, -0.000000000000000000 ) ) ;
#7951=DIRECTION ( 'NONE',  ( 0.000000000000000000, 0.000000000000000000, -1.000000000000000000 ) ) ;
#7976=AXIS2_PLACEMENT_3D ( 'NONE', #6552, #9621, #1872 ) ;
#7992=EDGE_CURVE ( 'NONE', #11981, #303, #4978, .T. ) ;
#8006=DIRECTION ( 'NONE',  ( -1.000000000000000000, -0.000000000000000000, -0.000000000000000000 ) ) ;
#8009=ORIENTED_EDGE ( 'NONE', *, *, #2548, .T. ) ;
#8014=DIRECTION ( 'NONE',  ( 1.000000000000000000, -0.000000000000000000, -0.000000000000000000 ) ) ;
#8020=AXIS2_PLACEMENT_3D ( 'NONE', #11516, #6785, #3720 ) ;
#8022=CARTESIAN_POINT ( 'NONE',  ( 36.00000000000000711, 0.000000000000000000, 0.000000000000000000 ) ) ;
#8031=DIRECTION ( 'NONE',  ( 0.000000000000000000, 0.000000000000000000, -1.000000000000000000 ) ) ;
#8044=DIRECTION ( 'NONE',  ( 0.000000000000000000, 0.000000000000000000, -1.000000000000000000 ) ) ;
#8045=VECTOR ( 'NONE', #6023, 1000.000000000000000 ) ;
#8052=EDGE_LOOP ( 'NONE', ( #5698, #2129, #508, #4803, #8142, #8793 ) ) ;
#8083=LINE ( 'NONE', #4184, #11762 ) ;
#8084=EDGE_CURVE ( 'NONE', #4496, #10589, #2383, .T. ) ;
#8085=CARTESIAN_POINT ( 'NONE',  ( -26.00000000000000355, 34.64101615137755630, 20.00000000000001066 ) ) ;
#8088=AXIS2_PLACEMENT_3D ( 'NONE', #4138, #5135, #8099 ) ;
#8094=AXIS2_PLACEMENT_3D ( 'NONE', #7147, #10945, #6395 ) ;
#8095=EDGE_LOOP ( 'NONE', ( #11257, #4078, #8643, #735 ) ) ;
#8097=LINE ( 'NONE', #10832, #8045 ) ;
#8098=ORIENTED_EDGE ( 'NONE', *, *, #10231, .F. ) ;
#8099=DIRECTION ( 'NONE',  ( 0.000000000000000000, 0.000000000000000000, -1.000000000000000000 ) ) ;
#8102=EDGE_CURVE ( 'NONE', #11745, #4049, #197, .T. ) ;
#8139=DIRECTION ( 'NONE',  ( 0.000000000000000000, 0.000000000000000000, 1.000000000000000000 ) ) ;
#8142=ORIENTED_EDGE ( 'NONE', *, *, #7444, .F. ) ;
#8154=FACE_OUTER_BOUND ( 'NONE', #7049, .T. ) ;
#8155=CARTESIAN_POINT ( 'NONE',  ( 36.00000000000000711, 34.64101615137756340, -19.99999999999998934 ) ) ;
#8215=CARTESIAN_POINT ( 'NONE',  ( 36.00000000000000711, 12.50000000000000000, -37.99671038392666134 ) ) ;
#8224=VECTOR ( 'NONE', #11140, 1000.000000000000000 ) ;
#8246=ORIENTED_EDGE ( 'NONE', *, *, #10117, .F. ) ;
#8269=DIRECTION ( 'NONE',  ( 0.000000000000000000, 0.000000000000000000, -1.000000000000000000 ) ) ;
#8270=DIRECTION ( 'NONE',  ( 0.000000000000000000, 0.000000000000000000, -1.000000000000000000 ) ) ;
#8284=DIRECTION ( 'NONE',  ( 1.000000000000000000, -0.000000000000000000, -0.000000000000000000 ) ) ;
#8289=VERTEX_POINT ( 'NONE', #1589 ) ;
#8298=DIRECTION ( 'NONE',  ( 0.000000000000000000, 0.000000000000000000, 1.000000000000000000 ) ) ;
#8318=CARTESIAN_POINT ( 'NONE',  ( 36.00000000000000000, 30.00000000000000711, 20.00000000000001066 ) ) ;
#8323=FILL_AREA_STYLE ('',( #6326 ) ) ;
#8341=ORIENTED_EDGE ( 'NONE', *, *, #5526, .F. ) ;
#8364=VECTOR ( 'NONE', #3675, 1000.000000000000000 ) ;
#8373=AXIS2_PLACEMENT_3D ( 'NONE', #8713, #6084, #9843 ) ;
#8378=CYLINDRICAL_SURFACE ( 'NONE', #10841, 7.500000000000000888 ) ;
#8382=DIRECTION ( 'NONE',  ( 0.000000000000000000, 0.000000000000000000, 1.000000000000000000 ) ) ;
#8386=EDGE_CURVE ( 'NONE', #6597, #6982, #8535, .T. ) ;
#8389=VECTOR ( 'NONE', #4001, 1000.000000000000000 ) ;
#8405=ORIENTED_EDGE ( 'NONE', *, *, #4945, .T. ) ;
#8417=VECTOR ( 'NONE', #7655, 1000.000000000000000 ) ;
#8422=CARTESIAN_POINT ( 'NONE',  ( -36.00000000000000711, 0.000000000000000000, 0.000000000000000000 ) ) ;
#8441=DIRECTION ( 'NONE',  ( 0.000000000000000000, 0.000000000000000000, -1.000000000000000000 ) ) ;
#8454=CARTESIAN_POINT ( 'NONE',  ( 33.00000000000000000, 6.368163355566238354E-16, -36.79999999999999716 ) ) ;
#8474=CARTESIAN_POINT ( 'NONE',  ( 26.00000000000000355, 0.000000000000000000, -41.99999999999999289 ) ) ;
#8475=VERTEX_POINT ( 'NONE', #2844 ) ;
#8480=DIRECTION ( 'NONE',  ( 0.000000000000000000, 0.000000000000000000, -1.000000000000000000 ) ) ;
#8485=FACE_OUTER_BOUND ( 'NONE', #5525, .T. ) ;
#8486=ORIENTED_EDGE ( 'NONE', *, *, #10306, .T. ) ;
#8492=AXIS2_PLACEMENT_3D ( 'NONE', #4638, #2748, #7711 ) ;
#8496=DIRECTION ( 'NONE',  ( 1.000000000000000000, -0.000000000000000000, -0.000000000000000000 ) ) ;
#8508=CARTESIAN_POINT ( 'NONE',  ( 26.00000000000000355, 0.000000000000000000, 0.000000000000000000 ) ) ;
#8517=EDGE_LOOP ( 'NONE', ( #8732, #1605 ) ) ;
#8518=LINE ( 'NONE', #131, #6385 ) ;
#8523=ORIENTED_EDGE ( 'NONE', *, *, #7992, .F. ) ;
#8535=LINE ( 'NONE', #10466, #10591 ) ;
#8536=PLANE ( 'NONE',  #8020 ) ;
#8569=ORIENTED_EDGE ( 'NONE', *, *, #10971, .T. ) ;
#8602=DIRECTION ( 'NONE',  ( 0.000000000000000000, 0.000000000000000000, -1.000000000000000000 ) ) ;
#8611=CARTESIAN_POINT ( 'NONE',  ( -36.00000000000000711, -4.898587196589413815E-15, -40.00000000000000711 ) ) ;
#8617=CARTESIAN_POINT ( 'NONE',  ( 36.00000000000000711, 0.000000000000000000, -7.500000000000000888 ) ) ;
#8624=CIRCLE ( 'NONE', #3422, 5.199999999999996625 ) ;
#8637=DIRECTION ( 'NONE',  ( 0.000000000000000000, 0.000000000000000000, -1.000000000000000000 ) ) ;
#8641=DIRECTION ( 'NONE',  ( 1.000000000000000000, -0.000000000000000000, -0.000000000000000000 ) ) ;
#8643=ORIENTED_EDGE ( 'NONE', *, *, #8979, .T. ) ;
#8652=DIRECTION ( 'NONE',  ( 0.000000000000000000, -0.000000000000000000, -1.000000000000000000 ) ) ;
#8658=VERTEX_POINT ( 'NONE', #12007 ) ;
#8669=EDGE_LOOP ( 'NONE', ( #10834, #12332, #8908, #983 ) ) ;
#8672=CARTESIAN_POINT ( 'NONE',  ( 36.00000000000000711, -12.50000000000000000, -24.50000000000000000 ) ) ;
#8676=VERTEX_POINT ( 'NONE', #3704 ) ;
#8680=CARTESIAN_POINT ( 'NONE',  ( 36.00000000000000711, 0.000000000000000000, -41.99999999999999289 ) ) ;
#8685=ORIENTED_EDGE ( 'NONE', *, *, #8913, .F. ) ;
#8692=AXIS2_PLACEMENT_3D ( 'NONE', #8474, #6588, #2836 ) ;
#8713=CARTESIAN_POINT ( 'NONE',  ( 36.00000000000000711, 0.000000000000000000, 0.000000000000000000 ) ) ;
#8716=EDGE_CURVE ( 'NONE', #2426, #6862, #9652, .T. ) ;
#8717=EDGE_LOOP ( 'NONE', ( #5577, #11851, #5481, #11332 ) ) ;
#8725=ORIENTED_EDGE ( 'NONE', *, *, #4901, .T. ) ;
#8731=ORIENTED_EDGE ( 'NONE', *, *, #6811, .T. ) ;
#8732=ORIENTED_EDGE ( 'NONE', *, *, #5315, .T. ) ;
#8733=EDGE_LOOP ( 'NONE', ( #1547, #5308, #4160, #5825 ) ) ;
#8753=DIRECTION ( 'NONE',  ( -0.000000000000000000, -0.000000000000000000, 1.000000000000000000 ) ) ;
#8757=DIRECTION ( 'NONE',  ( 0.000000000000000000, 0.000000000000000000, -1.000000000000000000 ) ) ;
#8782=EDGE_CURVE ( 'NONE', #2298, #1686, #213, .T. ) ;
#8787=AXIS2_PLACEMENT_3D ( 'NONE', #9889, #6949, #10750 ) ;
#8793=ORIENTED_EDGE ( 'NONE', *, *, #3900, .F. ) ;
#8800=DIRECTION ( 'NONE',  ( 1.000000000000000000, -0.000000000000000000, -0.000000000000000000 ) ) ;
#8805=ORIENTED_EDGE ( 'NONE', *, *, #3017, .T. ) ;
#8820=AXIS2_PLACEMENT_3D ( 'NONE', #4678, #9364, #11346 ) ;
#8826=CARTESIAN_POINT ( 'NONE',  ( 33.00000000000000000, 0.000000000000000000, 0.000000000000000000 ) ) ;
#8834=CIRCLE ( 'NONE', #4824, 40.00000000000000711 ) ;
#8846=CARTESIAN_POINT ( 'NONE',  ( -36.00000000000000000, 34.64101615137756340, -19.99999999999998934 ) ) ;
#8851=DIRECTION ( 'NONE',  ( 0.000000000000000000, 0.000000000000000000, 1.000000000000000000 ) ) ;
#8854=EDGE_CURVE ( 'NONE', #825, #11527, #2190, .T. ) ;
#8864=DIRECTION ( 'NONE',  ( 1.000000000000000000, 0.000000000000000000, 0.000000000000000000 ) ) ;
#8873=EDGE_LOOP ( 'NONE', ( #7598, #3204, #10, #9746 ) ) ;
#8894=DIRECTION ( 'NONE',  ( 1.000000000000000000, 0.000000000000000000, 0.000000000000000000 ) ) ;
#8901=DIRECTION ( 'NONE',  ( 1.000000000000000000, 0.000000000000000000, 0.000000000000000000 ) ) ;
#8903=VERTEX_POINT ( 'NONE', #8085 ) ;
#8907=SHAPE_REPRESENTATION ( 'main body', ( #6056 ), #6251 ) ;
#8908=ORIENTED_EDGE ( 'NONE', *, *, #10428, .F. ) ;
#8913=EDGE_CURVE ( 'NONE', #7918, #2661, #6612, .T. ) ;
#8914=DIRECTION ( 'NONE',  ( 0.000000000000000000, 0.000000000000000000, 1.000000000000000000 ) ) ;
#8947=CARTESIAN_POINT ( 'NONE',  ( 36.00000000000000711, 0.000000000000000000, 40.00000000000000711 ) ) ;
#8952=LINE ( 'NONE', #7839, #9606 ) ;
#8953=CARTESIAN_POINT ( 'NONE',  ( 36.00000000000000711, 0.000000000000000000, 0.000000000000000000 ) ) ;
#8960=FACE_OUTER_BOUND ( 'NONE', #2629, .T. ) ;
#8970=AXIS2_PLACEMENT_3D ( 'NONE', #4441, #1505, #8269 ) ;
#8973=ORIENTED_EDGE ( 'NONE', *, *, #790, .F. ) ;
#8979=EDGE_CURVE ( 'NONE', #3971, #825, #4627, .T. ) ;
#8988=ORIENTED_EDGE ( 'NONE', *, *, #4498, .T. ) ;
#9016=DIRECTION ( 'NONE',  ( 1.000000000000000000, 0.000000000000000000, 0.000000000000000000 ) ) ;
#9018=AXIS2_PLACEMENT_3D ( 'NONE', #5873, #162, #4340 ) ;
#9026=CARTESIAN_POINT ( 'NONE',  ( 36.00000000000000711, -12.50000000000000000, -37.99671038392666134 ) ) ;
#9046=ORIENTED_EDGE ( 'NONE', *, *, #10893, .T. ) ;
#9047=VECTOR ( 'NONE', #7901, 1000.000000000000000 ) ;
#9052=CARTESIAN_POINT ( 'NONE',  ( 33.00000000000000000, 0.000000000000000000, -49.49999999999999289 ) ) ;
#9059=DIRECTION ( 'NONE',  ( -1.000000000000000000, 0.000000000000000000, 0.000000000000000000 ) ) ;
#9067=VECTOR ( 'NONE', #8753, 1000.000000000000000 ) ;
#9074=EDGE_CURVE ( 'NONE', #11627, #451, #8624, .T. ) ;
#9097=FACE_OUTER_BOUND ( 'NONE', #5196, .T. ) ;
#9098=CIRCLE ( 'NONE', #1298, 6.500000000000000888 ) ;
#9124=CARTESIAN_POINT ( 'NONE',  ( -33.00000000000000000, -9.184850993605149917E-16, 7.500000000000000888 ) ) ;
#9125=EDGE_LOOP ( 'NONE', ( #4278, #8685, #10542, #7675 ) ) ;
#9128=CARTESIAN_POINT ( 'NONE',  ( -26.00000000000000355, 0.000000000000000000, 0.000000000000000000 ) ) ;
#9133=EDGE_CURVE ( 'NONE', #2147, #8289, #6979, .T. ) ;
#9142=ORIENTED_EDGE ( 'NONE', *, *, #9595, .T. ) ;
#9165=VECTOR ( 'NONE', #1877, 1000.000000000000000 ) ;
#9167=CARTESIAN_POINT ( 'NONE',  ( -36.00000000000000711, 34.64101615137755630, 20.00000000000001066 ) ) ;
#9168=AXIS2_PLACEMENT_3D ( 'NONE', #10368, #1810, #5625 ) ;
#9173=DIRECTION ( 'NONE',  ( 0.000000000000000000, 0.000000000000000000, -1.000000000000000000 ) ) ;
#9174=ORIENTED_EDGE ( 'NONE', *, *, #6629, .T. ) ;
#9189=EDGE_LOOP ( 'NONE', ( #6141, #11169, #1838, #6487 ) ) ;
#9213=VECTOR ( 'NONE', #6051, 1000.000000000000000 ) ;
#9253=ORIENTED_EDGE ( 'NONE', *, *, #11030, .F. ) ;
#9261=DIRECTION ( 'NONE',  ( 1.000000000000000000, -0.000000000000000000, -0.000000000000000000 ) ) ;
#9285=CARTESIAN_POINT ( 'NONE',  ( 15.00000000000000355, 40.00000000000000711, -1.999999999999998224 ) ) ;
#9300=CARTESIAN_POINT ( 'NONE',  ( 26.00000000000000355, 0.000000000000000000, -54.50000000000000000 ) ) ;
#9329=DIRECTION ( 'NONE',  ( 1.000000000000000000, 0.000000000000000000, 0.000000000000000000 ) ) ;
#9332=VERTEX_POINT ( 'NONE', #3480 ) ;
#9350=DIRECTION ( 'NONE',  ( -1.000000000000000000, -0.000000000000000000, -0.000000000000000000 ) ) ;
#9358=CARTESIAN_POINT ( 'NONE',  ( -15.00000000000000000, 40.00000000000000711, -2.000000000000000000 ) ) ;
#9364=DIRECTION ( 'NONE',  ( 1.000000000000000000, -0.000000000000000000, -0.000000000000000000 ) ) ;
#9408=AXIS2_PLACEMENT_3D ( 'NONE', #10128, #2547, #1796 ) ;
#9426=AXIS2_PLACEMENT_3D ( 'NONE', #1511, #3208, #5270 ) ;
#9430=VERTEX_POINT ( 'NONE', #10223 ) ;
#9435=ORIENTED_EDGE ( 'NONE', *, *, #6702, .T. ) ;
#9451=ADVANCED_FACE ( 'NONE', ( #6533 ), #5531, .F. ) ;
#9455=ORIENTED_EDGE ( 'NONE', *, *, #11725, .F. ) ;
#9476=ORIENTED_EDGE ( 'NONE', *, *, #9133, .F. ) ;
#9479=EDGE_CURVE ( 'NONE', #7148, #1686, #2659, .T. ) ;
#9482=DIRECTION ( 'NONE',  ( -1.000000000000000000, -0.000000000000000000, -0.000000000000000000 ) ) ;
#9487=EDGE_LOOP ( 'NONE', ( #1220, #8725, #11765, #8341 ) ) ;
#9492=DIRECTION ( 'NONE',  ( 1.000000000000000000, 0.000000000000000000, 0.000000000000000000 ) ) ;
#9502=AXIS2_PLACEMENT_3D ( 'NONE', #4495, #429, #7128 ) ;
#9511=ORIENTED_EDGE ( 'NONE', *, *, #11488, .T. ) ;
#9540=ORIENTED_EDGE ( 'NONE', *, *, #11134, .F. ) ;
#9545=ORIENTED_EDGE ( 'NONE', *, *, #9479, .F. ) ;
#9552=PLANE ( 'NONE',  #2418 ) ;
#9569=CARTESIAN_POINT ( 'NONE',  ( 33.00000000000000000, 0.000000000000000000, 0.000000000000000000 ) ) ;
#9575=CLOSED_SHELL ( 'NONE', ( #11410, #2182, #7463, #4939, #336, #6246, #12327, #3173, #11792, #5238, #7867, #7094, #11344, #5390, #9897, #7186, #1485, #7410, #663, #9451, #10215, #10229, #2354, #3554, #1437, #10455, #6780, #12247, #2935, #2552, #3354, #10267, #12089, #7269, #5037, #7541, #2173, #5567, #9708, #1869 ) ) ;
#9586=DIRECTION ( 'NONE',  ( 1.000000000000000000, -0.000000000000000000, -0.000000000000000000 ) ) ;
#9589=ORIENTED_EDGE ( 'NONE', *, *, #790, .T. ) ;
#9595=EDGE_CURVE ( 'NONE', #3450, #4147, #5027, .T. ) ;
#9603=ORIENTED_EDGE ( 'NONE', *, *, #7384, .F. ) ;
#9606=VECTOR ( 'NONE', #11634, 1000.000000000000000 ) ;
#9608=VECTOR ( 'NONE', #657, 1000.000000000000000 ) ;
#9621=DIRECTION ( 'NONE',  ( 1.000000000000000000, 0.000000000000000000, 0.000000000000000000 ) ) ;
#9624=ORIENTED_EDGE ( 'NONE', *, *, #11488, .F. ) ;
#9633=AXIS2_PLACEMENT_3D ( 'NONE', #1271, #10838, #8851 ) ;
#9634=FACE_OUTER_BOUND ( 'NONE', #3498, .T. ) ;
#9652=LINE ( 'NONE', #5900, #8417 ) ;
#9660=DIRECTION ( 'NONE',  ( 0.000000000000000000, 0.000000000000000000, -1.000000000000000000 ) ) ;
#9681=ORIENTED_EDGE ( 'NONE', *, *, #2140, .F. ) ;
#9691=ORIENTED_EDGE ( 'NONE', *, *, #3192, .F. ) ;
#9702=DIRECTION ( 'NONE',  ( -1.000000000000000000, 0.000000000000000000, 0.000000000000000000 ) ) ;
#9706=DIRECTION ( 'NONE',  ( 1.000000000000000000, 0.000000000000000000, 0.000000000000000000 ) ) ;
#9708=ADVANCED_FACE ( 'NONE', ( #8154 ), #5204, .F. ) ;
#9721=DIRECTION ( 'NONE',  ( 0.000000000000000000, 0.000000000000000000, -1.000000000000000000 ) ) ;
#9739=LINE ( 'NONE', #8611, #1218 ) ;
#9746=ORIENTED_EDGE ( 'NONE', *, *, #10305, .F. ) ;
#9749=PLANE ( 'NONE',  #3964 ) ;
#9764=CARTESIAN_POINT ( 'NONE',  ( 36.00000000000000000, 30.00000000000000711, 20.00000000000001066 ) ) ;
#9765=CIRCLE ( 'NONE', #6156, 40.00000000000000711 ) ;
#9768=CARTESIAN_POINT ( 'NONE',  ( 26.00000000000000355, 30.00000000000000711, 20.00000000000001066 ) ) ;
#9771=VERTEX_POINT ( 'NONE', #1521 ) ;
#9789=CYLINDRICAL_SURFACE ( 'NONE', #6230, 7.500000000000000888 ) ;
#9798=ORIENTED_EDGE ( 'NONE', *, *, #5463, .T. ) ;
#9802=CARTESIAN_POINT ( 'NONE',  ( -33.00000000000000000, 0.000000000000000000, -7.500000000000000888 ) ) ;
#9826=DIRECTION ( 'NONE',  ( 0.000000000000000000, 0.000000000000000000, -1.000000000000000000 ) ) ;
#9831=VECTOR ( 'NONE', #842, 1000.000000000000000 ) ;
#9843=DIRECTION ( 'NONE',  ( 0.000000000000000000, 0.000000000000000000, 1.000000000000000000 ) ) ;
#9847=ORIENTED_EDGE ( 'NONE', *, *, #1397, .T. ) ;
#9858=CARTESIAN_POINT ( 'NONE',  ( 26.00000000000000355, 0.000000000000000000, -34.49999999999999289 ) ) ;
#9873=DIRECTION ( 'NONE',  ( 1.000000000000000000, 0.000000000000000000, 0.000000000000000000 ) ) ;
#9880=DIRECTION ( 'NONE',  ( 0.000000000000000000, 0.000000000000000000, -1.000000000000000000 ) ) ;
#9889=CARTESIAN_POINT ( 'NONE',  ( -36.00000000000000711, 0.000000000000000000, 0.000000000000000000 ) ) ;
#9897=ADVANCED_FACE ( 'NONE', ( #12010, #7400, #3465 ), #7287, .F. ) ;
#9902=PRODUCT_DEFINITION_CONTEXT ( 'detailed design', #2570, 'design' ) ;
#9938=ORIENTED_EDGE ( 'NONE', *, *, #3411, .F. ) ;
#9943=DIRECTION ( 'NONE',  ( 0.000000000000000000, 0.000000000000000000, -1.000000000000000000 ) ) ;
#9946=FACE_OUTER_BOUND ( 'NONE', #2553, .T. ) ;
#9949=ORIENTED_EDGE ( 'NONE', *, *, #2334, .T. ) ;
#9952=ORIENTED_EDGE ( 'NONE', *, *, #2315, .F. ) ;
#9963=AXIS2_PLACEMENT_3D ( 'NONE', #8508, #5691, #8637 ) ;
#9978=CARTESIAN_POINT ( 'NONE',  ( -33.00000000000000000, 0.000000000000000000, 0.000000000000000000 ) ) ;
#9983=ORIENTED_EDGE ( 'NONE', *, *, #2803, .F. ) ;
#9986=VERTEX_POINT ( 'NONE', #5834 ) ;
#9995=ORIENTED_EDGE ( 'NONE', *, *, #3163, .F. ) ;
#10004=CARTESIAN_POINT ( 'NONE',  ( 36.00000000000000711, 12.50000000000000000, -37.99671038392666134 ) ) ;
#10011=FACE_BOUND ( 'NONE', #741, .T. ) ;
#10024=MECHANICAL_DESIGN_GEOMETRIC_PRESENTATION_REPRESENTATION('',(#11011),#10618);
#10061=EDGE_LOOP ( 'NONE', ( #10851, #3667, #6791, #9253 ) ) ;
#10065=DIRECTION ( 'NONE',  ( 1.000000000000000000, 0.000000000000000000, 0.000000000000000000 ) ) ;
#10069=EDGE_CURVE ( 'NONE', #11069, #8903, #10457, .T. ) ;
#10089=AXIS2_PLACEMENT_3D ( 'NONE', #1752, #3698, #2890 ) ;
#10096=CARTESIAN_POINT ( 'NONE',  ( 33.00000000000000000, 0.000000000000000000, -41.99999999999999289 ) ) ;
#10097=VECTOR ( 'NONE', #6257, 1000.000000000000000 ) ;
#10098=EDGE_CURVE ( 'NONE', #9771, #11527, #5257, .T. ) ;
#10108=CARTESIAN_POINT ( 'NONE',  ( -26.00000000000000355, -7.960204194457796463E-16, -6.500000000000000888 ) ) ;
#10114=DIRECTION ( 'NONE',  ( 1.000000000000000000, 0.000000000000000000, 0.000000000000000000 ) ) ;
#10117=EDGE_CURVE ( 'NONE', #5845, #11069, #1447, .T. ) ;
#10128=CARTESIAN_POINT ( 'NONE',  ( 15.00000000000000355, 40.00000000000000711, 0.000000000000000000 ) ) ;
#10166=CIRCLE ( 'NONE', #4772, 7.500000000000000888 ) ;
#10167=DIRECTION ( 'NONE',  ( 0.000000000000000000, 0.000000000000000000, -1.000000000000000000 ) ) ;
#10172=ORIENTED_EDGE ( 'NONE', *, *, #10879, .F. ) ;
#10177=EDGE_LOOP ( 'NONE', ( #11857, #9798, #11934, #10263 ) ) ;
#10185=EDGE_LOOP ( 'NONE', ( #9603, #1550, #8009, #6659 ) ) ;
#10187=DIRECTION ( 'NONE',  ( 0.000000000000000000, 0.000000000000000000, 1.000000000000000000 ) ) ;
#10213=ORIENTED_EDGE ( 'NONE', *, *, #11975, .T. ) ;
#10215=ADVANCED_FACE ( 'NONE', ( #2311, #9946, #3374 ), #5128, .T. ) ;
#10223=CARTESIAN_POINT ( 'NONE',  ( 15.00000000000000355, 30.00000000000000711, -1.999999999999998224 ) ) ;
#10229=ADVANCED_FACE ( 'NONE', ( #3448 ), #8378, .F. ) ;
#10231=EDGE_CURVE ( 'NONE', #1934, #5929, #2440, .T. ) ;
#10232=PRODUCT_DEFINITION_FORMATION_WITH_SPECIFIED_SOURCE ( 'ANY', '', #6127, .NOT_KNOWN. ) ;
#10235=CYLINDRICAL_SURFACE ( 'NONE', #1164, 12.49999999999999645 ) ;
#10241=DIRECTION ( 'NONE',  ( 0.000000000000000000, 0.000000000000000000, -1.000000000000000000 ) ) ;
#10263=ORIENTED_EDGE ( 'NONE', *, *, #4246, .F. ) ;
#10267=ADVANCED_FACE ( 'NONE', ( #739 ), #12109, .T. ) ;
#10300=DIRECTION ( 'NONE',  ( 0.000000000000000000, -1.000000000000000000, 0.000000000000000000 ) ) ;
#10303=ORIENTED_EDGE ( 'NONE', *, *, #4945, .F. ) ;
#10305=EDGE_CURVE ( 'NONE', #10589, #2426, #1166, .T. ) ;
#10306=EDGE_CURVE ( 'NONE', #103, #5845, #11119, .T. ) ;
#10319=VERTEX_POINT ( 'NONE', #4365 ) ;
#10329=( LENGTH_UNIT ( ) NAMED_UNIT ( * ) SI_UNIT ( .MILLI., .METRE. ) );
#10331=FACE_BOUND ( 'NONE', #5817, .T. ) ;
#10335=ORIENTED_EDGE ( 'NONE', *, *, #8979, .F. ) ;
#10350=EDGE_LOOP ( 'NONE', ( #9681, #4849, #4427, #6920 ) ) ;
#10366=DIRECTION ( 'NONE',  ( 1.000000000000000000, 0.000000000000000000, 0.000000000000000000 ) ) ;
#10368=CARTESIAN_POINT ( 'NONE',  ( 15.00000000000000355, 30.00000000000000711, 0.000000000000000000 ) ) ;
#10384=ORIENTED_EDGE ( 'NONE', *, *, #8782, .F. ) ;
#10392=DIRECTION ( 'NONE',  ( 1.000000000000000000, -0.000000000000000000, -0.000000000000000000 ) ) ;
#10399=DIRECTION ( 'NONE',  ( 0.000000000000000000, 0.000000000000000000, -1.000000000000000000 ) ) ;
#10416=EDGE_LOOP ( 'NONE', ( #3024, #5250 ) ) ;
#10428=EDGE_CURVE ( 'NONE', #3761, #4605, #3575, .T. ) ;
#10432=ORIENTED_EDGE ( 'NONE', *, *, #11883, .F. ) ;
#10433=LINE ( 'NONE', #7698, #9165 ) ;
#10446=DIRECTION ( 'NONE',  ( -1.000000000000000000, 0.000000000000000000, 0.000000000000000000 ) ) ;
#10455=ADVANCED_FACE ( 'NONE', ( #2936, #7754 ), #10498, .F. ) ;
#10457=LINE ( 'NONE', #3014, #4855 ) ;
#10466=CARTESIAN_POINT ( 'NONE',  ( 15.00000000000000355, 40.00000000000000711, 1.999999999999998224 ) ) ;
#10497=EDGE_CURVE ( 'NONE', #6597, #9430, #5767, .T. ) ;
#10498=PLANE ( 'NONE',  #11340 ) ;
#10511=CARTESIAN_POINT ( 'NONE',  ( 26.00000000000000355, -12.50000000000000000, -41.99999999999999289 ) ) ;
#10527=ORIENTED_EDGE ( 'NONE', *, *, #4860, .F. ) ;
#10529=DIRECTION ( 'NONE',  ( 1.000000000000000000, -0.000000000000000000, -0.000000000000000000 ) ) ;
#10542=ORIENTED_EDGE ( 'NONE', *, *, #5526, .T. ) ;
#10550=DIRECTION ( 'NONE',  ( 1.000000000000000000, -0.000000000000000000, -0.000000000000000000 ) ) ;
#10555=CARTESIAN_POINT ( 'NONE',  ( -26.00000000000000355, 0.000000000000000000, 0.000000000000000000 ) ) ;
#10586=FACE_OUTER_BOUND ( 'NONE', #8052, .T. ) ;
#10589=VERTEX_POINT ( 'NONE', #2243 ) ;
#10591=VECTOR ( 'NONE', #19, 1000.000000000000000 ) ;
#10593=LINE ( 'NONE', #11405, #12050 ) ;
#10609=VECTOR ( 'NONE', #11288, 1000.000000000000000 ) ;
#10618=( GEOMETRIC_REPRESENTATION_CONTEXT ( 3 ) GLOBAL_UNCERTAINTY_ASSIGNED_CONTEXT ( ( #1655 ) ) GLOBAL_UNIT_ASSIGNED_CONTEXT ( ( #6454, #1694, #6380 ) ) REPRESENTATION_CONTEXT ( 'NONE', 'WORKASPACE' ) );
#10639=VERTEX_POINT ( 'NONE', #5997 ) ;
#10648=FACE_OUTER_BOUND ( 'NONE', #10350, .T. ) ;
#10673=DIRECTION ( 'NONE',  ( 1.000000000000000000, 0.000000000000000000, 0.000000000000000000 ) ) ;
#10679=EDGE_CURVE ( 'NONE', #8903, #3376, #6574, .T. ) ;
#10685=CIRCLE ( 'NONE', #8492, 5.199999999999996625 ) ;
#10718=FACE_OUTER_BOUND ( 'NONE', #4108, .T. ) ;
#10735=EDGE_CURVE ( 'NONE', #709, #4941, #5172, .T. ) ;
#10750=DIRECTION ( 'NONE',  ( 0.000000000000000000, 0.000000000000000000, 1.000000000000000000 ) ) ;
#10759=CYLINDRICAL_SURFACE ( 'NONE', #8373, 40.00000000000000711 ) ;
#10764=VERTEX_POINT ( 'NONE', #3614 ) ;
#10765=DIRECTION ( 'NONE',  ( 1.000000000000000000, -0.000000000000000000, -0.000000000000000000 ) ) ;
#10766=AXIS2_PLACEMENT_3D ( 'NONE', #9128, #9261, #10241 ) ;
#10774=DIRECTION ( 'NONE',  ( 0.000000000000000000, 1.000000000000000000, 0.000000000000000000 ) ) ;
#10786=CARTESIAN_POINT ( 'NONE',  ( 33.00000000000000000, 7.960204194457796463E-16, -6.500000000000000888 ) ) ;
#10806=AXIS2_PLACEMENT_3D ( 'NONE', #2758, #12075, #6585 ) ;
#10818=PRODUCT_DEFINITION_SHAPE ( 'NONE', 'NONE',  #3130 ) ;
#10832=CARTESIAN_POINT ( 'NONE',  ( 36.00000000000000000, 40.00000000000000711, -19.99999999999998934 ) ) ;
#10833=AXIS2_PLACEMENT_3D ( 'NONE', #10896, #6146, #8914 ) ;
#10834=ORIENTED_EDGE ( 'NONE', *, *, #807, .T. ) ;
#10838=DIRECTION ( 'NONE',  ( 1.000000000000000000, -0.000000000000000000, -0.000000000000000000 ) ) ;
#10841=AXIS2_PLACEMENT_3D ( 'NONE', #7328, #7273, #7508 ) ;
#10851=ORIENTED_EDGE ( 'NONE', *, *, #1051, .F. ) ;
#10855=DIRECTION ( 'NONE',  ( 0.000000000000000000, 0.000000000000000000, -1.000000000000000000 ) ) ;
#10860=CARTESIAN_POINT ( 'NONE',  ( -13.05124837953327344, 0.000000000000000000, -41.99999999999999289 ) ) ;
#10872=CIRCLE ( 'NONE', #8692, 12.49999999999999645 ) ;
#10879=EDGE_CURVE ( 'NONE', #231, #4639, #188, .T. ) ;
#10887=CARTESIAN_POINT ( 'NONE',  ( 36.00000000000000711, 0.000000000000000000, 6.500000000000000888 ) ) ;
#10891=ORIENTED_EDGE ( 'NONE', *, *, #7267, .T. ) ;
#10893=EDGE_CURVE ( 'NONE', #5929, #9771, #11554, .T. ) ;
#10896=CARTESIAN_POINT ( 'NONE',  ( 15.00000000000000355, 40.00000000000000711, 0.000000000000000000 ) ) ;
#10908=LINE ( 'NONE', #9802, #9213 ) ;
#10928=CYLINDRICAL_SURFACE ( 'NONE', #596, 7.500000000000000888 ) ;
#10930=FACE_OUTER_BOUND ( 'NONE', #8733, .T. ) ;
#10931=DIRECTION ( 'NONE',  ( 0.000000000000000000, 0.000000000000000000, -1.000000000000000000 ) ) ;
#10938=DIRECTION ( 'NONE',  ( -1.000000000000000000, -0.000000000000000000, -0.000000000000000000 ) ) ;
#10939=ORIENTED_EDGE ( 'NONE', *, *, #12053, .T. ) ;
#10942=CYLINDRICAL_SURFACE ( 'NONE', #9633, 6.500000000000000888 ) ;
#10945=DIRECTION ( 'NONE',  ( -0.000000000000000000, 1.000000000000000000, -0.000000000000000000 ) ) ;
#10954=FACE_OUTER_BOUND ( 'NONE', #9189, .T. ) ;
#10971=EDGE_CURVE ( 'NONE', #4639, #231, #10166, .T. ) ;
#10976=VECTOR ( 'NONE', #10366, 1000.000000000000000 ) ;
#10988=VECTOR ( 'NONE', #9016, 1000.000000000000000 ) ;
#11001=DIRECTION ( 'NONE',  ( 1.000000000000000000, 0.000000000000000000, 0.000000000000000000 ) ) ;
#11004=VERTEX_POINT ( 'NONE', #1331 ) ;
#11009=EDGE_LOOP ( 'NONE', ( #4343, #7091 ) ) ;
#11011=STYLED_ITEM ( 'NONE', ( #11924 ), #4209 ) ;
#11020=CARTESIAN_POINT ( 'NONE',  ( -36.00000000000000711, 0.000000000000000000, 0.000000000000000000 ) ) ;
#11022=CIRCLE ( 'NONE', #2642, 7.500000000000000888 ) ;
#11024=LINE ( 'NONE', #2461, #12134 ) ;
#11030=EDGE_CURVE ( 'NONE', #5880, #11004, #1417, .T. ) ;
#11033=VECTOR ( 'NONE', #7055, 1000.000000000000000 ) ;
#11043=ORIENTED_EDGE ( 'NONE', *, *, #11030, .T. ) ;
#11059=FACE_OUTER_BOUND ( 'NONE', #8717, .T. ) ;
#11067=DIRECTION ( 'NONE',  ( -0.000000000000000000, -1.000000000000000000, -0.000000000000000000 ) ) ;
#11069=VERTEX_POINT ( 'NONE', #5339 ) ;
#11071=CARTESIAN_POINT ( 'NONE',  ( 26.00000000000000355, 0.000000000000000000, 40.00000000000000711 ) ) ;
#11077=ORIENTED_EDGE ( 'NONE', *, *, #10069, .F. ) ;
#11081=CYLINDRICAL_SURFACE ( 'NONE', #8094, 2.000000000000000000 ) ;
#11097=CARTESIAN_POINT ( 'NONE',  ( 26.00000000000000355, 34.64101615137756340, -19.99999999999998934 ) ) ;
#11118=DIRECTION ( 'NONE',  ( -1.000000000000000000, 0.000000000000000000, 0.000000000000000000 ) ) ;
#11119=LINE ( 'NONE', #5447, #971 ) ;
#11125=SURFACE_STYLE_USAGE ( .BOTH. , #3453 ) ;
#11134=EDGE_CURVE ( 'NONE', #11902, #8475, #3828, .T. ) ;
#11138=EDGE_LOOP ( 'NONE', ( #6355, #1758, #57, #10891 ) ) ;
#11140=DIRECTION ( 'NONE',  ( 0.000000000000000000, -1.000000000000000000, 0.000000000000000000 ) ) ;
#11145=EDGE_LOOP ( 'NONE', ( #11659, #2676 ) ) ;
#11169=ORIENTED_EDGE ( 'NONE', *, *, #10735, .F. ) ;
#11173=AXIS2_PLACEMENT_3D ( 'NONE', #2400, #3297, #11843 ) ;
#11191=AXIS2_PLACEMENT_3D ( 'NONE', #5146, #7222, #11601 ) ;
#11192=EDGE_CURVE ( 'NONE', #12066, #103, #3712, .T. ) ;
#11201=CARTESIAN_POINT ( 'NONE',  ( 36.00000000000000000, 30.00000000000000711, 20.00000000000001066 ) ) ;
#11203=ORIENTED_EDGE ( 'NONE', *, *, #1397, .F. ) ;
#11232=DIRECTION ( 'NONE',  ( 0.000000000000000000, 0.000000000000000000, 1.000000000000000000 ) ) ;
#11234=ORIENTED_EDGE ( 'NONE', *, *, #7002, .T. ) ;
#11238=CIRCLE ( 'NONE', #5863, 1.999999999999998224 ) ;
#11244=DIRECTION ( 'NONE',  ( 0.000000000000000000, 0.000000000000000000, -1.000000000000000000 ) ) ;
#11257=ORIENTED_EDGE ( 'NONE', *, *, #10098, .F. ) ;
#11267=CARTESIAN_POINT ( 'NONE',  ( -15.00000000000000000, 40.00000000000000711, 0.000000000000000000 ) ) ;
#11288=DIRECTION ( 'NONE',  ( -0.000000000000000000, 1.000000000000000000, -0.000000000000000000 ) ) ;
#11289=CYLINDRICAL_SURFACE ( 'NONE', #11351, 7.500000000000000000 ) ;
#11303=CARTESIAN_POINT ( 'NONE',  ( 33.00000000000000000, 0.000000000000000000, -41.99999999999999289 ) ) ;
#11327=CARTESIAN_POINT ( 'NONE',  ( 26.00000000000000355, 9.184850993605147944E-16, -49.49999999999999289 ) ) ;
#11332=ORIENTED_EDGE ( 'NONE', *, *, #11725, .T. ) ;
#11340=AXIS2_PLACEMENT_3D ( 'NONE', #10555, #9702, #6642 ) ;
#11344=ADVANCED_FACE ( 'NONE', ( #7772 ), #2085, .F. ) ;
#11346=DIRECTION ( 'NONE',  ( 0.000000000000000000, 0.000000000000000000, 1.000000000000000000 ) ) ;
#11347=FACE_OUTER_BOUND ( 'NONE', #11145, .T. ) ;
#11351=AXIS2_PLACEMENT_3D ( 'NONE', #969, #4788, #11232 ) ;
#11355=ORIENTED_EDGE ( 'NONE', *, *, #12267, .T. ) ;
#11402=DIRECTION ( 'NONE',  ( 1.000000000000000000, -0.000000000000000000, -0.000000000000000000 ) ) ;
#11405=CARTESIAN_POINT ( 'NONE',  ( -36.00000000000000000, 30.00000000000000711, -19.99999999999998934 ) ) ;
#11410=ADVANCED_FACE ( 'NONE', ( #7845 ), #11641, .F. ) ;
#11476=CARTESIAN_POINT ( 'NONE',  ( -26.00000000000000355, 0.000000000000000000, 0.000000000000000000 ) ) ;
#11488=EDGE_CURVE ( 'NONE', #8676, #12066, #5028, .T. ) ;
#11489=EDGE_CURVE ( 'NONE', #10639, #3355, #8097, .T. ) ;
#11510=LINE ( 'NONE', #4836, #96 ) ;
#11511=UNCERTAINTY_MEASURE_WITH_UNIT (LENGTH_MEASURE( 1.000000000000000082E-05 ), #2556, 'distance_accuracy_value', 'NONE');
#11516=CARTESIAN_POINT ( 'NONE',  ( -36.00000000000000000, 0.000000000000000000, 0.000000000000000000 ) ) ;
#11524=ORIENTED_EDGE ( 'NONE', *, *, #6811, .F. ) ;
#11526=ORIENTED_EDGE ( 'NONE', *, *, #430, .F. ) ;
#11527=VERTEX_POINT ( 'NONE', #9026 ) ;
#11544=ORIENTED_EDGE ( 'NONE', *, *, #1051, .T. ) ;
#11550=EDGE_CURVE ( 'NONE', #5230, #3761, #4191, .T. ) ;
#11554=CIRCLE ( 'NONE', #7976, 40.00000000000000711 ) ;
#11557=DIRECTION ( 'NONE',  ( -1.000000000000000000, 0.000000000000000000, 0.000000000000000000 ) ) ;
#11576=DIRECTION ( 'NONE',  ( -1.000000000000000000, 0.000000000000000000, -0.000000000000000000 ) ) ;
#11595=AXIS2_PLACEMENT_3D ( 'NONE', #9978, #9059, #294 ) ;
#11601=DIRECTION ( 'NONE',  ( 0.000000000000000000, 0.000000000000000000, -1.000000000000000000 ) ) ;
#11602=EDGE_LOOP ( 'NONE', ( #10527, #3352, #6310, #1542 ) ) ;
#11614=DIRECTION ( 'NONE',  ( -1.000000000000000000, -0.000000000000000000, -0.000000000000000000 ) ) ;
#11617=AXIS2_PLACEMENT_3D ( 'NONE', #10860, #6112, #9173 ) ;
#11626=DIRECTION ( 'NONE',  ( 0.000000000000000000, 0.000000000000000000, 1.000000000000000000 ) ) ;
#11627=VERTEX_POINT ( 'NONE', #8454 ) ;
#11634=DIRECTION ( 'NONE',  ( -0.000000000000000000, 0.000000000000000000, 1.000000000000000000 ) ) ;
#11641=CYLINDRICAL_SURFACE ( 'NONE', #3840, 2.000000000000000000 ) ;
#11659=ORIENTED_EDGE ( 'NONE', *, *, #4021, .T. ) ;
#11697=FACE_OUTER_BOUND ( 'NONE', #4014, .T. ) ;
#11725=EDGE_CURVE ( 'NONE', #1709, #1424, #1840, .T. ) ;
#11745=VERTEX_POINT ( 'NONE', #7708 ) ;
#11751=DIRECTION ( 'NONE',  ( 1.000000000000000000, 0.000000000000000000, 0.000000000000000000 ) ) ;
#11762=VECTOR ( 'NONE', #8014, 1000.000000000000000 ) ;
#11765=ORIENTED_EDGE ( 'NONE', *, *, #5315, .F. ) ;
#11789=VECTOR ( 'NONE', #9350, 1000.000000000000000 ) ;
#11792=ADVANCED_FACE ( 'NONE', ( #2887 ), #2073, .F. ) ;
#11805=DIRECTION ( 'NONE',  ( -1.000000000000000000, -0.000000000000000000, -0.000000000000000000 ) ) ;
#11806=EDGE_LOOP ( 'NONE', ( #1232, #12072, #3468, #10335, #2479, #9476, #9938, #3398, #9624, #8805 ) ) ;
#11811=CARTESIAN_POINT ( 'NONE',  ( 36.00000000000000711, 0.000000000000000000, 0.000000000000000000 ) ) ;
#11823=CIRCLE ( 'NONE', #12205, 2.000000000000000000 ) ;
#11829=DIRECTION ( 'NONE',  ( 1.000000000000000000, -0.000000000000000000, -0.000000000000000000 ) ) ;
#11843=DIRECTION ( 'NONE',  ( 0.000000000000000000, 0.000000000000000000, 1.000000000000000000 ) ) ;
#11851=ORIENTED_EDGE ( 'NONE', *, *, #4021, .F. ) ;
#11855=CARTESIAN_POINT ( 'NONE',  ( 36.00000000000000000, 40.00000000000000711, 20.00000000000001066 ) ) ;
#11856=EDGE_CURVE ( 'NONE', #1686, #2298, #11022, .T. ) ;
#11857=ORIENTED_EDGE ( 'NONE', *, *, #2651, .F. ) ;
#11883=EDGE_CURVE ( 'NONE', #4951, #11004, #2303, .T. ) ;
#11890=ORIENTED_EDGE ( 'NONE', *, *, #3900, .T. ) ;
#11902=VERTEX_POINT ( 'NONE', #3190 ) ;
#11910=CARTESIAN_POINT ( 'NONE',  ( 33.00000000000000000, 0.000000000000000000, -41.99999999999999289 ) ) ;
#11923=CARTESIAN_POINT ( 'NONE',  ( 29.00000000000000000, 0.000000000000000000, -41.99999999999999289 ) ) ;
#11924=PRESENTATION_STYLE_ASSIGNMENT (( #11125 ) ) ;
#11934=ORIENTED_EDGE ( 'NONE', *, *, #11550, .T. ) ;
#11938=DIRECTION ( 'NONE',  ( -1.000000000000000000, -0.000000000000000000, -0.000000000000000000 ) ) ;
#11975=EDGE_CURVE ( 'NONE', #8289, #5929, #1248, .T. ) ;
#11981=VERTEX_POINT ( 'NONE', #10108 ) ;
#11984=APPLICATION_CONTEXT ( 'automotive_design' ) ;
#11990=VECTOR ( 'NONE', #6690, 1000.000000000000000 ) ;
#11993=CARTESIAN_POINT ( 'NONE',  ( -33.00000000000000000, 0.000000000000000000, 0.000000000000000000 ) ) ;
#12000=CARTESIAN_POINT ( 'NONE',  ( 33.00000000000000000, 0.000000000000000000, 6.500000000000000888 ) ) ;
#12007=CARTESIAN_POINT ( 'NONE',  ( 33.00000000000000000, 0.000000000000000000, -7.500000000000000888 ) ) ;
#12010=FACE_BOUND ( 'NONE', #4113, .T. ) ;
#12012=AXIS2_PLACEMENT_3D ( 'NONE', #9569, #8641, #6709 ) ;
#12015=DIRECTION ( 'NONE',  ( 1.000000000000000000, -0.000000000000000000, -0.000000000000000000 ) ) ;
#12050=VECTOR ( 'NONE', #1152, 1000.000000000000000 ) ;
#12053=EDGE_CURVE ( 'NONE', #4049, #11745, #11823, .T. ) ;
#12066=VERTEX_POINT ( 'NONE', #11097 ) ;
#12072=ORIENTED_EDGE ( 'NONE', *, *, #4860, .T. ) ;
#12074=VECTOR ( 'NONE', #10300, 1000.000000000000000 ) ;
#12075=DIRECTION ( 'NONE',  ( 1.000000000000000000, -0.000000000000000000, -0.000000000000000000 ) ) ;
#12089=ADVANCED_FACE ( 'NONE', ( #1594 ), #3238, .T. ) ;
#12092=LINE ( 'NONE', #6117, #1035 ) ;
#12099=EDGE_LOOP ( 'NONE', ( #10384, #2160 ) ) ;
#12102=EDGE_CURVE ( 'NONE', #11745, #10319, #589, .T. ) ;
#12109=PLANE ( 'NONE',  #5454 ) ;
#12110=DIRECTION ( 'NONE',  ( 0.000000000000000000, -1.000000000000000000, 0.000000000000000000 ) ) ;
#12134=VECTOR ( 'NONE', #6660, 1000.000000000000000 ) ;
#12147=VECTOR ( 'NONE', #5357, 1000.000000000000000 ) ;
#12157=EDGE_CURVE ( 'NONE', #1491, #6982, #12221, .T. ) ;
#12163=ORIENTED_EDGE ( 'NONE', *, *, #396, .F. ) ;
#12171=FACE_BOUND ( 'NONE', #3940, .T. ) ;
#12185=VECTOR ( 'NONE', #1478, 1000.000000000000000 ) ;
#12196=ORIENTED_EDGE ( 'NONE', *, *, #10971, .F. ) ;
#12205=AXIS2_PLACEMENT_3D ( 'NONE', #7115, #1535, #5351 ) ;
#12208=VECTOR ( 'NONE', #5519, 1000.000000000000000 ) ;
#12221=CIRCLE ( 'NONE', #2821, 1.999999999999998224 ) ;
#12235=CARTESIAN_POINT ( 'NONE',  ( -36.00000000000000711, 0.000000000000000000, 0.000000000000000000 ) ) ;
#12247=ADVANCED_FACE ( 'NONE', ( #8485 ), #2851, .F. ) ;
#12267=EDGE_CURVE ( 'NONE', #2661, #7918, #2450, .T. ) ;
#12294=CARTESIAN_POINT ( 'NONE',  ( -26.00000000000000355, 30.00000000000000711, -19.99999999999998934 ) ) ;
#12321=CARTESIAN_POINT ( 'NONE',  ( 36.00000000000000000, 30.00000000000000711, 20.00000000000001066 ) ) ;
#12327=ADVANCED_FACE ( 'NONE', ( #10718 ), #3966, .T. ) ;
#12332=ORIENTED_EDGE ( 'NONE', *, *, #2651, .T. ) ;
#12345=CARTESIAN_POINT ( 'NONE',  ( 36.00000000000000711, 12.50000000000000000, -41.99999999999999289 ) ) ;
#12371=COLOUR_RGB('Dark Blue',0.08,0.2,0.34);
#12372=FILL_AREA_STYLE_COLOUR('',#12371);
#12373=FILL_AREA_STYLE('',(#12372));
#12374=SURFACE_STYLE_FILL_AREA(#12373);
#12375=SURFACE_SIDE_STYLE('',(#12374));
#12376=SURFACE_STYLE_USAGE(.BOTH.,#12375);
#12377=PRESENTATION_STYLE_ASSIGNMENT((#12376));
ENDSEC;
END-ISO-10303-21;
